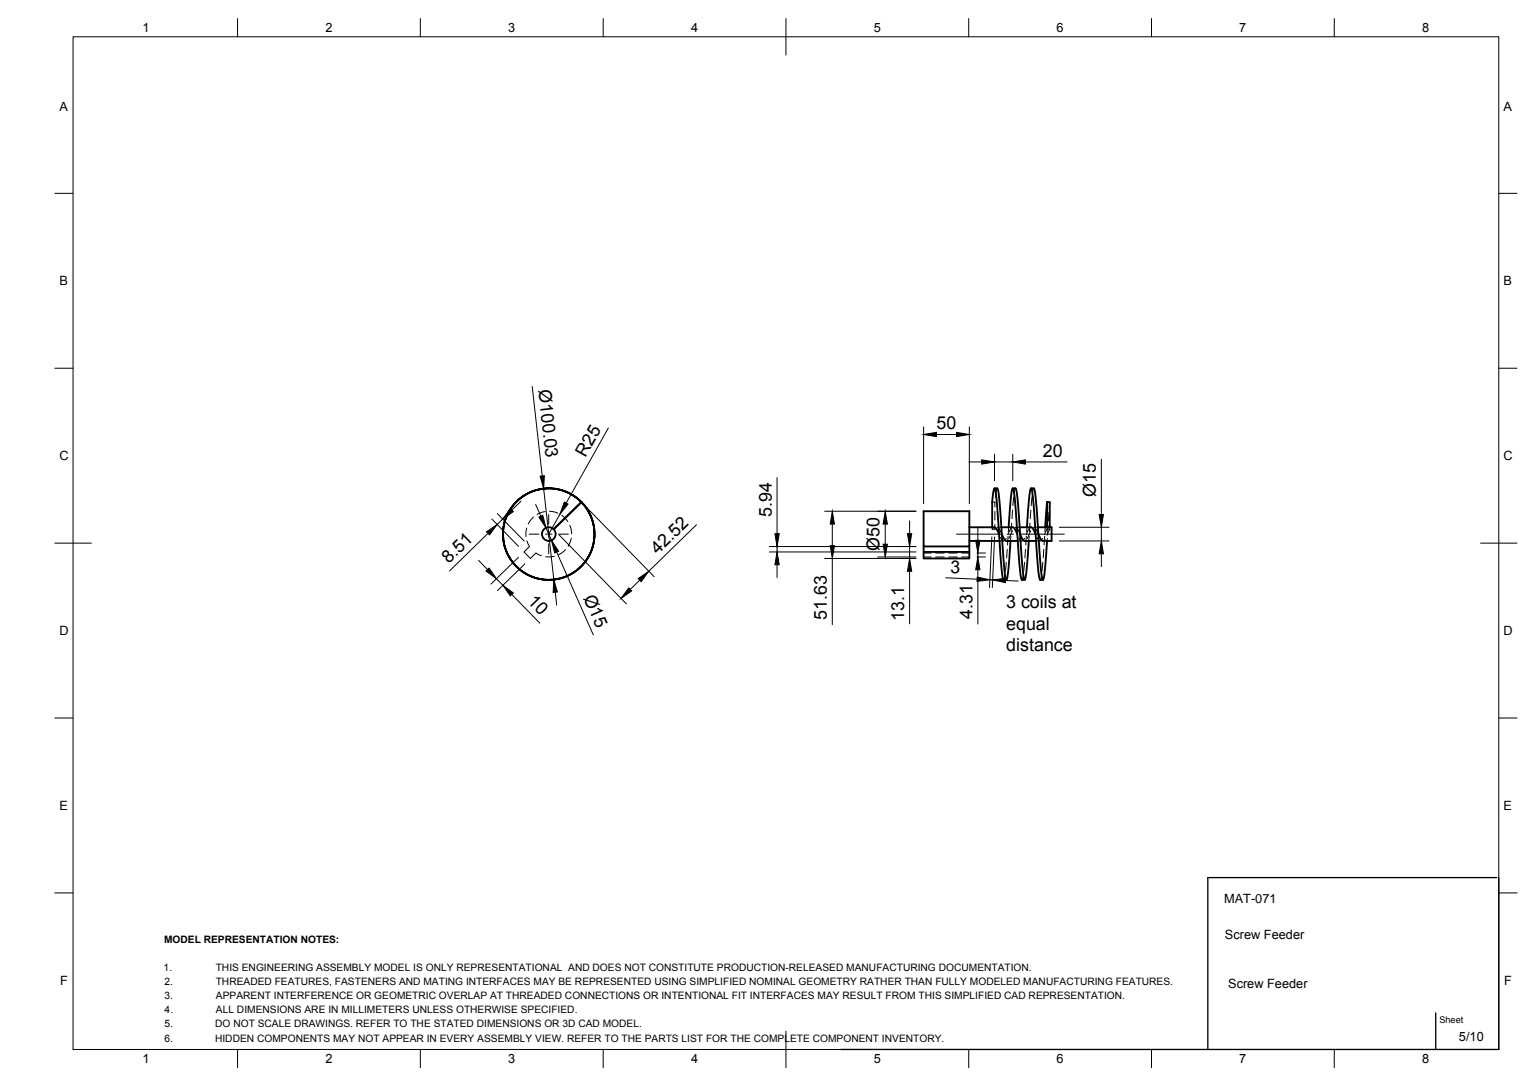
ISO-10303-21;
HEADER;
/* Generated by software containing ST-Developer
 * from STEP Tools, Inc. (www.steptools.com) 
 */

FILE_DESCRIPTION(
/* description */ (''),
/* implementation_level */ '2;1');

FILE_NAME(
/* name */ 'Screw Feeder.step',
/* time_stamp */ '2026-10-24T12:24:47-07:00',
/* author */ (''),
/* organization */ (''),
/* preprocessor_version */ 'ST-DEVELOPER v20.2',
/* originating_system */ 'Autodesk Translation Framework v15.15.0.0',
/* authorisation */ '');

FILE_SCHEMA (('AUTOMOTIVE_DESIGN { 1 0 10303 214 3 1 1 }'));
ENDSEC;

DATA;
#10=MECHANICAL_DESIGN_GEOMETRIC_PRESENTATION_REPRESENTATION('',(#62),#13594);
#50=SHAPE_REPRESENTATION_RELATIONSHIP('SRR','None',#13630,#56);
#56=ADVANCED_BREP_SHAPE_REPRESENTATION('',(#68),#13593);
#62=STYLED_ITEM('',(#13667),#68);
#68=MANIFOLD_SOLID_BREP('Screw Feeder',#2969);
#71=(
BOUNDED_SURFACE()
B_SPLINE_SURFACE(1,2,((#12578,#12579,#12580,#12581,#12582,#12583,#12584,
#12585,#12586,#12587,#12588,#12589,#12590,#12591,#12592,#12593,#12594,#12595,
#12596,#12597,#12598,#12599,#12600,#12601,#12602,#12603,#12604,#12605,#12606,
#12607,#12608,#12609,#12610,#12611,#12612,#12613,#12614,#12615,#12616,#12617,
#12618,#12619,#12620,#12621,#12622,#12623,#12624,#12625,#12626,#12627,#12628,
#12629,#12630,#12631,#12632,#12633,#12634,#12635,#12636,#12637,#12638,#12639,
#12640,#12641,#12642,#12643,#12644,#12645,#12646,#12647,#12648,#12649,#12650,
#12651,#12652,#12653,#12654,#12655,#12656,#12657,#12658,#12659,#12660,#12661,
#12662,#12663,#12664,#12665,#12666,#12667,#12668,#12669,#12670,#12671,#12672,
#12673,#12674,#12675,#12676,#12677,#12678,#12679,#12680,#12681,#12682,#12683,
#12684,#12685,#12686,#12687,#12688,#12689,#12690,#12691,#12692,#12693,#12694,
#12695,#12696,#12697,#12698),(#12699,#12700,#12701,#12702,#12703,#12704,
#12705,#12706,#12707,#12708,#12709,#12710,#12711,#12712,#12713,#12714,#12715,
#12716,#12717,#12718,#12719,#12720,#12721,#12722,#12723,#12724,#12725,#12726,
#12727,#12728,#12729,#12730,#12731,#12732,#12733,#12734,#12735,#12736,#12737,
#12738,#12739,#12740,#12741,#12742,#12743,#12744,#12745,#12746,#12747,#12748,
#12749,#12750,#12751,#12752,#12753,#12754,#12755,#12756,#12757,#12758,#12759,
#12760,#12761,#12762,#12763,#12764,#12765,#12766,#12767,#12768,#12769,#12770,
#12771,#12772,#12773,#12774,#12775,#12776,#12777,#12778,#12779,#12780,#12781,
#12782,#12783,#12784,#12785,#12786,#12787,#12788,#12789,#12790,#12791,#12792,
#12793,#12794,#12795,#12796,#12797,#12798,#12799,#12800,#12801,#12802,#12803,
#12804,#12805,#12806,#12807,#12808,#12809,#12810,#12811,#12812,#12813,#12814,
#12815,#12816,#12817,#12818,#12819)),.UNSPECIFIED.,.F.,.F.,.F.)
B_SPLINE_SURFACE_WITH_KNOTS((2,2),(3,2,2,2,2,2,2,2,2,2,2,2,2,2,2,2,2,2,
2,2,2,2,2,2,2,2,2,2,2,2,2,2,2,2,2,2,2,2,2,2,2,2,2,2,2,2,2,2,2,2,2,2,2,2,
2,2,2,2,2,2,3),(0.,1.),(0.,0.0166666666666667,0.0333333333333333,0.05,0.0666666666666667,
0.0833333333333333,0.1,0.116666666666667,0.133333333333333,0.15,0.166666666666667,
0.183333333333333,0.2,0.216666666666667,0.233333333333333,0.25,0.266666666666667,
0.283333333333333,0.3,0.316666666666667,0.333333333333333,0.35,0.366666666666667,
0.383333333333333,0.4,0.416666666666667,0.433333333333333,0.45,0.466666666666667,
0.483333333333333,0.5,0.516666666666667,0.533333333333333,0.55,0.566666666666667,
0.583333333333333,0.6,0.616666666666667,0.633333333333333,0.65,0.666666666666667,
0.683333333333333,0.7,0.716666666666667,0.733333333333333,0.75,0.766666666666667,
0.783333333333333,0.8,0.816666666666667,0.833333333333333,0.85,0.866666666666667,
0.883333333333333,0.9,0.916666666666667,0.933333333333333,0.95,0.966666666666667,
0.983333333333333,1.),.UNSPECIFIED.)
GEOMETRIC_REPRESENTATION_ITEM()
RATIONAL_B_SPLINE_SURFACE(((1.,0.987688340595138,1.,0.987688340595138,1.,
0.987688340595138,1.,0.987688340595138,1.,0.987688340595138,1.,0.987688340595138,
1.,0.987688340595138,1.,0.987688340595138,1.,0.987688340595138,1.,0.987688340595138,
1.,0.987688340595138,1.,0.987688340595138,1.,0.987688340595138,1.,0.987688340595138,
1.,0.987688340595138,1.,0.987688340595138,1.,0.987688340595138,1.,0.987688340595138,
1.,0.987688340595138,1.,0.987688340595138,1.,0.987688340595138,1.,0.987688340595138,
1.,0.987688340595138,1.,0.987688340595138,1.,0.987688340595138,1.,0.987688340595138,
1.,0.987688340595138,1.,0.987688340595138,1.,0.987688340595138,1.,0.987688340595138,
1.,0.987688340595138,1.,0.987688340595138,1.,0.987688340595138,1.,0.987688340595138,
1.,0.987688340595138,1.,0.987688340595138,1.,0.987688340595138,1.,0.987688340595138,
1.,0.987688340595138,1.,0.987688340595138,1.,0.987688340595138,1.,0.987688340595138,
1.,0.987688340595138,1.,0.987688340595138,1.,0.987688340595138,1.,0.987688340595138,
1.,0.987688340595138,1.,0.987688340595138,1.,0.987688340595138,1.,0.987688340595138,
1.,0.987688340595138,1.,0.987688340595138,1.,0.987688340595138,1.,0.987688340595138,
1.,0.987688340595138,1.,0.987688340595138,1.,0.987688340595138,1.,0.987688340595138,
1.,0.987688340595138,1.,0.987688340595138,1.),(1.,0.987688340595138,1.,
0.987688340595138,1.,0.987688340595138,1.,0.987688340595138,1.,0.987688340595138,
1.,0.987688340595138,1.,0.987688340595138,1.,0.987688340595138,1.,0.987688340595138,
1.,0.987688340595138,1.,0.987688340595138,1.,0.987688340595138,1.,0.987688340595138,
1.,0.987688340595138,1.,0.987688340595138,1.,0.987688340595138,1.,0.987688340595138,
1.,0.987688340595138,1.,0.987688340595138,1.,0.987688340595138,1.,0.987688340595138,
1.,0.987688340595138,1.,0.987688340595138,1.,0.987688340595138,1.,0.987688340595138,
1.,0.987688340595138,1.,0.987688340595138,1.,0.987688340595138,1.,0.987688340595138,
1.,0.987688340595138,1.,0.987688340595138,1.,0.987688340595138,1.,0.987688340595138,
1.,0.987688340595138,1.,0.987688340595138,1.,0.987688340595138,1.,0.987688340595138,
1.,0.987688340595138,1.,0.987688340595138,1.,0.987688340595138,1.,0.987688340595138,
1.,0.987688340595138,1.,0.987688340595138,1.,0.987688340595138,1.,0.987688340595138,
1.,0.987688340595138,1.,0.987688340595138,1.,0.987688340595138,1.,0.987688340595138,
1.,0.987688340595138,1.,0.987688340595138,1.,0.987688340595138,1.,0.987688340595138,
1.,0.987688340595138,1.,0.987688340595138,1.,0.987688340595138,1.,0.987688340595138,
1.,0.987688340595138,1.,0.987688340595138,1.,0.987688340595138,1.)))
REPRESENTATION_ITEM('')
SURFACE()
);
#72=(
BOUNDED_SURFACE()
B_SPLINE_SURFACE(1,2,((#12941,#12942,#12943,#12944,#12945,#12946,#12947,
#12948,#12949,#12950,#12951,#12952,#12953,#12954,#12955,#12956,#12957,#12958,
#12959,#12960,#12961,#12962,#12963,#12964,#12965,#12966,#12967,#12968,#12969,
#12970,#12971,#12972,#12973,#12974,#12975,#12976,#12977,#12978,#12979,#12980,
#12981,#12982,#12983,#12984,#12985,#12986,#12987,#12988,#12989,#12990,#12991,
#12992,#12993,#12994,#12995,#12996,#12997,#12998,#12999,#13000,#13001,#13002,
#13003,#13004,#13005,#13006,#13007,#13008,#13009,#13010,#13011,#13012,#13013,
#13014,#13015,#13016,#13017,#13018,#13019,#13020,#13021,#13022,#13023,#13024,
#13025,#13026,#13027,#13028,#13029,#13030,#13031,#13032,#13033,#13034,#13035,
#13036,#13037,#13038,#13039,#13040,#13041,#13042,#13043,#13044,#13045,#13046,
#13047,#13048,#13049,#13050,#13051,#13052,#13053,#13054,#13055,#13056,#13057,
#13058,#13059,#13060,#13061),(#13062,#13063,#13064,#13065,#13066,#13067,
#13068,#13069,#13070,#13071,#13072,#13073,#13074,#13075,#13076,#13077,#13078,
#13079,#13080,#13081,#13082,#13083,#13084,#13085,#13086,#13087,#13088,#13089,
#13090,#13091,#13092,#13093,#13094,#13095,#13096,#13097,#13098,#13099,#13100,
#13101,#13102,#13103,#13104,#13105,#13106,#13107,#13108,#13109,#13110,#13111,
#13112,#13113,#13114,#13115,#13116,#13117,#13118,#13119,#13120,#13121,#13122,
#13123,#13124,#13125,#13126,#13127,#13128,#13129,#13130,#13131,#13132,#13133,
#13134,#13135,#13136,#13137,#13138,#13139,#13140,#13141,#13142,#13143,#13144,
#13145,#13146,#13147,#13148,#13149,#13150,#13151,#13152,#13153,#13154,#13155,
#13156,#13157,#13158,#13159,#13160,#13161,#13162,#13163,#13164,#13165,#13166,
#13167,#13168,#13169,#13170,#13171,#13172,#13173,#13174,#13175,#13176,#13177,
#13178,#13179,#13180,#13181,#13182)),.UNSPECIFIED.,.F.,.F.,.F.)
B_SPLINE_SURFACE_WITH_KNOTS((2,2),(3,2,2,2,2,2,2,2,2,2,2,2,2,2,2,2,2,2,
2,2,2,2,2,2,2,2,2,2,2,2,2,2,2,2,2,2,2,2,2,2,2,2,2,2,2,2,2,2,2,2,2,2,2,2,
2,2,2,2,2,2,3),(0.,1.),(0.,0.0166666666666667,0.0333333333333333,0.05,0.0666666666666667,
0.0833333333333333,0.1,0.116666666666667,0.133333333333333,0.15,0.166666666666667,
0.183333333333333,0.2,0.216666666666667,0.233333333333333,0.25,0.266666666666667,
0.283333333333333,0.3,0.316666666666667,0.333333333333333,0.35,0.366666666666667,
0.383333333333333,0.4,0.416666666666667,0.433333333333333,0.45,0.466666666666667,
0.483333333333333,0.5,0.516666666666667,0.533333333333333,0.55,0.566666666666667,
0.583333333333333,0.6,0.616666666666667,0.633333333333333,0.65,0.666666666666667,
0.683333333333333,0.7,0.716666666666667,0.733333333333333,0.75,0.766666666666667,
0.783333333333333,0.8,0.816666666666667,0.833333333333333,0.85,0.866666666666667,
0.883333333333333,0.9,0.916666666666667,0.933333333333333,0.95,0.966666666666667,
0.983333333333333,1.),.UNSPECIFIED.)
GEOMETRIC_REPRESENTATION_ITEM()
RATIONAL_B_SPLINE_SURFACE(((1.,0.987688340595138,1.,0.987688340595138,1.,
0.987688340595138,1.,0.987688340595138,1.,0.987688340595138,1.,0.987688340595138,
1.,0.987688340595138,1.,0.987688340595138,1.,0.987688340595138,1.,0.987688340595138,
1.,0.987688340595138,1.,0.987688340595138,1.,0.987688340595138,1.,0.987688340595138,
1.,0.987688340595138,1.,0.987688340595138,1.,0.987688340595138,1.,0.987688340595138,
1.,0.987688340595138,1.,0.987688340595138,1.,0.987688340595138,1.,0.987688340595138,
1.,0.987688340595138,1.,0.987688340595138,1.,0.987688340595138,1.,0.987688340595138,
1.,0.987688340595138,1.,0.987688340595138,1.,0.987688340595138,1.,0.987688340595138,
1.,0.987688340595138,1.,0.987688340595138,1.,0.987688340595138,1.,0.987688340595138,
1.,0.987688340595138,1.,0.987688340595138,1.,0.987688340595138,1.,0.987688340595138,
1.,0.987688340595138,1.,0.987688340595138,1.,0.987688340595138,1.,0.987688340595138,
1.,0.987688340595138,1.,0.987688340595138,1.,0.987688340595138,1.,0.987688340595138,
1.,0.987688340595138,1.,0.987688340595138,1.,0.987688340595138,1.,0.987688340595138,
1.,0.987688340595138,1.,0.987688340595138,1.,0.987688340595138,1.,0.987688340595138,
1.,0.987688340595138,1.,0.987688340595138,1.,0.987688340595138,1.,0.987688340595138,
1.,0.987688340595138,1.,0.987688340595138,1.),(1.,0.987688340595138,1.,
0.987688340595138,1.,0.987688340595138,1.,0.987688340595138,1.,0.987688340595138,
1.,0.987688340595138,1.,0.987688340595138,1.,0.987688340595138,1.,0.987688340595138,
1.,0.987688340595138,1.,0.987688340595138,1.,0.987688340595138,1.,0.987688340595138,
1.,0.987688340595138,1.,0.987688340595138,1.,0.987688340595138,1.,0.987688340595138,
1.,0.987688340595138,1.,0.987688340595138,1.,0.987688340595138,1.,0.987688340595138,
1.,0.987688340595138,1.,0.987688340595138,1.,0.987688340595138,1.,0.987688340595138,
1.,0.987688340595138,1.,0.987688340595138,1.,0.987688340595138,1.,0.987688340595138,
1.,0.987688340595138,1.,0.987688340595138,1.,0.987688340595138,1.,0.987688340595138,
1.,0.987688340595138,1.,0.987688340595138,1.,0.987688340595138,1.,0.987688340595138,
1.,0.987688340595138,1.,0.987688340595138,1.,0.987688340595138,1.,0.987688340595138,
1.,0.987688340595138,1.,0.987688340595138,1.,0.987688340595138,1.,0.987688340595138,
1.,0.987688340595138,1.,0.987688340595138,1.,0.987688340595138,1.,0.987688340595138,
1.,0.987688340595138,1.,0.987688340595138,1.,0.987688340595138,1.,0.987688340595138,
1.,0.987688340595138,1.,0.987688340595138,1.,0.987688340595138,1.,0.987688340595138,
1.,0.987688340595138,1.,0.987688340595138,1.,0.987688340595138,1.)))
REPRESENTATION_ITEM('')
SURFACE()
);
#73=(
BOUNDED_SURFACE()
B_SPLINE_SURFACE(1,2,((#13304,#13305,#13306,#13307,#13308,#13309,#13310,
#13311,#13312,#13313,#13314,#13315,#13316,#13317,#13318,#13319,#13320,#13321,
#13322,#13323,#13324,#13325,#13326,#13327,#13328,#13329,#13330,#13331,#13332,
#13333,#13334,#13335,#13336,#13337,#13338,#13339,#13340,#13341,#13342,#13343,
#13344,#13345,#13346,#13347,#13348,#13349,#13350,#13351,#13352,#13353,#13354,
#13355,#13356,#13357,#13358,#13359,#13360,#13361,#13362,#13363,#13364,#13365,
#13366,#13367,#13368,#13369,#13370,#13371,#13372,#13373,#13374,#13375,#13376,
#13377,#13378,#13379,#13380,#13381,#13382,#13383,#13384,#13385,#13386,#13387,
#13388,#13389,#13390,#13391,#13392,#13393,#13394,#13395,#13396,#13397,#13398,
#13399,#13400,#13401,#13402,#13403,#13404,#13405,#13406,#13407,#13408,#13409,
#13410,#13411,#13412,#13413,#13414,#13415,#13416,#13417,#13418,#13419,#13420,
#13421,#13422,#13423,#13424),(#13425,#13426,#13427,#13428,#13429,#13430,
#13431,#13432,#13433,#13434,#13435,#13436,#13437,#13438,#13439,#13440,#13441,
#13442,#13443,#13444,#13445,#13446,#13447,#13448,#13449,#13450,#13451,#13452,
#13453,#13454,#13455,#13456,#13457,#13458,#13459,#13460,#13461,#13462,#13463,
#13464,#13465,#13466,#13467,#13468,#13469,#13470,#13471,#13472,#13473,#13474,
#13475,#13476,#13477,#13478,#13479,#13480,#13481,#13482,#13483,#13484,#13485,
#13486,#13487,#13488,#13489,#13490,#13491,#13492,#13493,#13494,#13495,#13496,
#13497,#13498,#13499,#13500,#13501,#13502,#13503,#13504,#13505,#13506,#13507,
#13508,#13509,#13510,#13511,#13512,#13513,#13514,#13515,#13516,#13517,#13518,
#13519,#13520,#13521,#13522,#13523,#13524,#13525,#13526,#13527,#13528,#13529,
#13530,#13531,#13532,#13533,#13534,#13535,#13536,#13537,#13538,#13539,#13540,
#13541,#13542,#13543,#13544,#13545)),.UNSPECIFIED.,.F.,.F.,.F.)
B_SPLINE_SURFACE_WITH_KNOTS((2,2),(3,2,2,2,2,2,2,2,2,2,2,2,2,2,2,2,2,2,
2,2,2,2,2,2,2,2,2,2,2,2,2,2,2,2,2,2,2,2,2,2,2,2,2,2,2,2,2,2,2,2,2,2,2,2,
2,2,2,2,2,2,3),(0.,1.),(0.,0.0166666666666667,0.0333333333333333,0.05,0.0666666666666667,
0.0833333333333333,0.1,0.116666666666667,0.133333333333333,0.15,0.166666666666667,
0.183333333333333,0.2,0.216666666666667,0.233333333333333,0.25,0.266666666666667,
0.283333333333333,0.3,0.316666666666667,0.333333333333333,0.35,0.366666666666667,
0.383333333333333,0.4,0.416666666666667,0.433333333333333,0.45,0.466666666666667,
0.483333333333333,0.5,0.516666666666667,0.533333333333333,0.55,0.566666666666667,
0.583333333333333,0.6,0.616666666666667,0.633333333333333,0.65,0.666666666666667,
0.683333333333333,0.7,0.716666666666667,0.733333333333333,0.75,0.766666666666667,
0.783333333333333,0.8,0.816666666666667,0.833333333333333,0.85,0.866666666666667,
0.883333333333333,0.9,0.916666666666667,0.933333333333333,0.95,0.966666666666667,
0.983333333333333,1.),.UNSPECIFIED.)
GEOMETRIC_REPRESENTATION_ITEM()
RATIONAL_B_SPLINE_SURFACE(((1.,0.987688340595138,1.,0.987688340595138,1.,
0.987688340595138,1.,0.987688340595138,1.,0.987688340595138,1.,0.987688340595138,
1.,0.987688340595138,1.,0.987688340595138,1.,0.987688340595138,1.,0.987688340595138,
1.,0.987688340595138,1.,0.987688340595138,1.,0.987688340595138,1.,0.987688340595138,
1.,0.987688340595138,1.,0.987688340595138,1.,0.987688340595138,1.,0.987688340595138,
1.,0.987688340595138,1.,0.987688340595138,1.,0.987688340595138,1.,0.987688340595138,
1.,0.987688340595138,1.,0.987688340595138,1.,0.987688340595138,1.,0.987688340595138,
1.,0.987688340595138,1.,0.987688340595138,1.,0.987688340595138,1.,0.987688340595138,
1.,0.987688340595138,1.,0.987688340595138,1.,0.987688340595138,1.,0.987688340595138,
1.,0.987688340595138,1.,0.987688340595138,1.,0.987688340595138,1.,0.987688340595138,
1.,0.987688340595138,1.,0.987688340595138,1.,0.987688340595138,1.,0.987688340595138,
1.,0.987688340595138,1.,0.987688340595138,1.,0.987688340595138,1.,0.987688340595138,
1.,0.987688340595138,1.,0.987688340595138,1.,0.987688340595138,1.,0.987688340595138,
1.,0.987688340595138,1.,0.987688340595138,1.,0.987688340595138,1.,0.987688340595138,
1.,0.987688340595138,1.,0.987688340595138,1.,0.987688340595138,1.,0.987688340595138,
1.,0.987688340595138,1.,0.987688340595138,1.),(1.,0.987688340595138,1.,
0.987688340595138,1.,0.987688340595138,1.,0.987688340595138,1.,0.987688340595138,
1.,0.987688340595138,1.,0.987688340595138,1.,0.987688340595138,1.,0.987688340595138,
1.,0.987688340595138,1.,0.987688340595138,1.,0.987688340595138,1.,0.987688340595138,
1.,0.987688340595138,1.,0.987688340595138,1.,0.987688340595138,1.,0.987688340595138,
1.,0.987688340595138,1.,0.987688340595138,1.,0.987688340595138,1.,0.987688340595138,
1.,0.987688340595138,1.,0.987688340595138,1.,0.987688340595138,1.,0.987688340595138,
1.,0.987688340595138,1.,0.987688340595138,1.,0.987688340595138,1.,0.987688340595138,
1.,0.987688340595138,1.,0.987688340595138,1.,0.987688340595138,1.,0.987688340595138,
1.,0.987688340595138,1.,0.987688340595138,1.,0.987688340595138,1.,0.987688340595138,
1.,0.987688340595138,1.,0.987688340595138,1.,0.987688340595138,1.,0.987688340595138,
1.,0.987688340595138,1.,0.987688340595138,1.,0.987688340595138,1.,0.987688340595138,
1.,0.987688340595138,1.,0.987688340595138,1.,0.987688340595138,1.,0.987688340595138,
1.,0.987688340595138,1.,0.987688340595138,1.,0.987688340595138,1.,0.987688340595138,
1.,0.987688340595138,1.,0.987688340595138,1.,0.987688340595138,1.,0.987688340595138,
1.,0.987688340595138,1.,0.987688340595138,1.,0.987688340595138,1.)))
REPRESENTATION_ITEM('')
SURFACE()
);
#104=PLANE('',#3260);
#105=PLANE('',#3261);
#106=PLANE('',#3262);
#107=PLANE('',#3266);
#108=PLANE('',#3267);
#109=PLANE('',#3268);
#110=PLANE('',#3269);
#111=PLANE('',#3270);
#134=FACE_BOUND('',#568,.T.);
#143=B_SPLINE_CURVE_WITH_KNOTS('',3,(#11375,#11376,#11377,#11378),
 .UNSPECIFIED.,.F.,.F.,(4,4),(-1.,-0.998645968698766),.UNSPECIFIED.);
#144=B_SPLINE_CURVE_WITH_KNOTS('',3,(#11385,#11386,#11387,#11388,#11389,
#11390,#11391,#11392,#11393,#11394,#11395,#11396,#11397,#11398,#11399,#11400,
#11401,#11402,#11403,#11404,#11405,#11406,#11407,#11408,#11409,#11410,#11411,
#11412,#11413,#11414,#11415,#11416,#11417,#11418,#11419,#11420,#11421,#11422,
#11423,#11424,#11425,#11426,#11427,#11428,#11429,#11430,#11431,#11432,#11433,
#11434,#11435,#11436,#11437,#11438,#11439,#11440,#11441,#11442,#11443,#11444,
#11445,#11446,#11447,#11448,#11449,#11450,#11451,#11452,#11453,#11454,#11455,
#11456,#11457,#11458,#11459,#11460,#11461,#11462,#11463,#11464,#11465,#11466,
#11467,#11468,#11469,#11470,#11471,#11472,#11473,#11474,#11475,#11476,#11477,
#11478,#11479,#11480,#11481,#11482,#11483,#11484,#11485,#11486,#11487,#11488,
#11489,#11490,#11491,#11492,#11493,#11494,#11495,#11496,#11497,#11498,#11499,
#11500,#11501,#11502,#11503,#11504,#11505,#11506,#11507,#11508,#11509,#11510,
#11511,#11512,#11513,#11514,#11515,#11516,#11517,#11518,#11519,#11520,#11521,
#11522,#11523,#11524,#11525,#11526,#11527,#11528,#11529,#11530,#11531,#11532,
#11533,#11534,#11535,#11536,#11537,#11538,#11539,#11540,#11541,#11542,#11543,
#11544,#11545,#11546,#11547,#11548,#11549,#11550,#11551,#11552,#11553,#11554,
#11555,#11556,#11557,#11558,#11559,#11560,#11561,#11562,#11563,#11564,#11565,
#11566,#11567,#11568,#11569,#11570,#11571,#11572,#11573,#11574,#11575,#11576,
#11577,#11578,#11579,#11580,#11581,#11582,#11583,#11584,#11585,#11586,#11587,
#11588,#11589,#11590,#11591,#11592,#11593,#11594,#11595,#11596,#11597,#11598,
#11599,#11600,#11601,#11602,#11603,#11604,#11605,#11606,#11607,#11608,#11609,
#11610,#11611,#11612,#11613,#11614,#11615,#11616,#11617,#11618,#11619,#11620,
#11621,#11622,#11623,#11624,#11625,#11626,#11627,#11628,#11629,#11630,#11631,
#11632,#11633,#11634,#11635,#11636,#11637,#11638,#11639,#11640,#11641,#11642,
#11643,#11644,#11645,#11646,#11647,#11648,#11649,#11650,#11651,#11652,#11653,
#11654,#11655,#11656,#11657,#11658,#11659,#11660,#11661,#11662,#11663,#11664,
#11665,#11666,#11667,#11668,#11669,#11670,#11671,#11672,#11673,#11674,#11675,
#11676,#11677,#11678,#11679,#11680,#11681,#11682,#11683,#11684,#11685,#11686,
#11687,#11688,#11689,#11690,#11691,#11692,#11693,#11694,#11695,#11696,#11697,
#11698,#11699,#11700,#11701,#11702,#11703,#11704,#11705,#11706,#11707,#11708,
#11709,#11710,#11711,#11712,#11713,#11714,#11715,#11716,#11717,#11718,#11719,
#11720,#11721,#11722,#11723,#11724,#11725,#11726,#11727,#11728,#11729,#11730,
#11731,#11732,#11733,#11734,#11735,#11736,#11737,#11738,#11739,#11740,#11741,
#11742),.UNSPECIFIED.,.F.,.F.,(4,3,3,3,3,3,3,3,3,3,3,3,3,3,3,3,3,3,3,3,
3,3,3,3,3,3,3,3,3,3,3,3,3,3,3,3,3,3,3,3,3,3,3,3,3,3,3,3,3,3,3,3,3,3,3,3,
3,3,3,3,3,3,3,3,3,3,3,3,3,3,3,3,3,3,3,3,3,3,3,3,3,3,3,3,3,3,3,3,3,3,3,3,
3,3,3,3,3,3,3,3,3,3,3,3,3,3,3,3,3,3,3,3,3,3,3,3,3,3,3,4),(-0.331979302032099,
-0.328745544947817,-0.325511126349503,-0.322277581756429,-0.319042795051795,
-0.316666666666667,-0.313432410645245,-0.310074307983934,-0.306840488099785,
-0.303607230746873,-0.300373105768056,-0.3,-0.296765743978578,-0.293407641317267,
-0.290173821433118,-0.286940564080179,-0.283706439101408,-0.283333333333333,
-0.280099077311897,-0.27674097465059,-0.273507154766441,-0.270273897413541,
-0.267039772434759,-0.266666666666667,-0.263432410645244,-0.260074307983933,
-0.25684048809978,-0.253607230746841,-0.250373105768036,-0.25,-0.246765743978575,
-0.243407641317264,-0.240173821433105,-0.236940564080198,-0.233706439101398,
-0.233333333333333,-0.230099077311924,-0.22674097465061,-0.223507154766454,
-0.220273897413536,-0.217039772434708,-0.216666666666667,-0.213432410645268,
-0.210074307983951,-0.206840488099798,-0.203607230746877,-0.200373105768084,
-0.2,-0.196765743978578,-0.193407641317267,-0.190173821433123,-0.186940564080229,
-0.183706439101414,-0.183333333333333,-0.180099077311908,-0.176740974650597,
-0.173507154766428,-0.170273897413483,-0.167039772434678,-0.166666666666667,
-0.163432410645259,-0.160074307983944,-0.156840488099797,-0.153607230746853,
-0.150373105768069,-0.15,-0.146765743978574,-0.143407641317264,-0.140173821433101,
-0.136940564080169,-0.133706439101386,-0.133333333333333,-0.130099077311911,
-0.1267409746506,-0.123507154766447,-0.120273897413526,-0.117039772434722,
-0.116666666666667,-0.113432410645241,-0.110074307983931,-0.106840488099774,
-0.103607230746858,-0.10037310576804,-0.1,-0.0967657439785776,-0.0934076413172665,
-0.0901738214331063,-0.0869405640801917,-0.0837064391013879,-0.0833333333333334,
-0.0800990773119075,-0.0767409746505973,-0.0735071547664396,-0.0702738974135466,
-0.0670397724347522,-0.0666666666666667,-0.0634324106452447,-0.0600743079839336,
-0.0568404880997839,-0.0536072307468639,-0.0503731057680767,-0.05,-0.0467657439785748,
-0.0434076413172644,-0.0401738214331216,-0.0369405640801967,-0.033706439101418,
-0.0333333333333333,-0.030099077311911,-0.0267409746505999,-0.0235071547664523,
-0.0202738974135343,-0.017039772434738,-0.0166666666666667,-0.0134324106517174,
-0.0100743318149406,-0.00684051195133032,-0.00360725461687006,-0.000373129688631168,
-9.53046099950368E-8),.UNSPECIFIED.);
#145=B_SPLINE_CURVE_WITH_KNOTS('',3,(#11789,#11790,#11791,#11792,#11793,
#11794,#11795,#11796,#11797,#11798,#11799,#11800,#11801,#11802,#11803,#11804,
#11805,#11806,#11807,#11808,#11809,#11810,#11811,#11812,#11813,#11814,#11815,
#11816,#11817,#11818,#11819,#11820,#11821,#11822,#11823,#11824,#11825,#11826,
#11827,#11828,#11829,#11830,#11831,#11832,#11833,#11834,#11835,#11836,#11837,
#11838,#11839,#11840,#11841,#11842,#11843,#11844,#11845,#11846,#11847,#11848,
#11849,#11850,#11851,#11852,#11853,#11854,#11855,#11856,#11857,#11858,#11859,
#11860,#11861,#11862,#11863,#11864,#11865,#11866,#11867,#11868,#11869,#11870,
#11871,#11872,#11873,#11874,#11875,#11876,#11877,#11878,#11879,#11880,#11881,
#11882,#11883,#11884,#11885,#11886,#11887,#11888,#11889,#11890,#11891,#11892,
#11893,#11894,#11895,#11896,#11897,#11898,#11899,#11900,#11901,#11902,#11903,
#11904,#11905,#11906,#11907,#11908,#11909,#11910,#11911,#11912,#11913,#11914,
#11915,#11916,#11917,#11918,#11919,#11920,#11921,#11922,#11923,#11924,#11925,
#11926,#11927,#11928,#11929,#11930,#11931,#11932,#11933,#11934,#11935,#11936,
#11937,#11938,#11939,#11940,#11941,#11942,#11943,#11944,#11945,#11946,#11947,
#11948,#11949,#11950,#11951,#11952,#11953,#11954,#11955,#11956,#11957,#11958,
#11959,#11960,#11961,#11962,#11963,#11964,#11965,#11966,#11967,#11968,#11969,
#11970,#11971,#11972,#11973,#11974,#11975,#11976,#11977,#11978,#11979,#11980,
#11981,#11982,#11983,#11984,#11985,#11986,#11987,#11988,#11989,#11990,#11991,
#11992,#11993,#11994,#11995,#11996,#11997,#11998,#11999,#12000,#12001,#12002,
#12003,#12004,#12005,#12006,#12007,#12008,#12009,#12010,#12011,#12012,#12013,
#12014,#12015,#12016,#12017,#12018,#12019,#12020,#12021,#12022,#12023,#12024,
#12025,#12026,#12027,#12028,#12029,#12030,#12031,#12032,#12033,#12034,#12035,
#12036,#12037,#12038,#12039,#12040,#12041,#12042,#12043,#12044,#12045,#12046,
#12047,#12048,#12049,#12050,#12051,#12052,#12053,#12054,#12055,#12056,#12057,
#12058,#12059,#12060,#12061,#12062,#12063,#12064,#12065,#12066,#12067,#12068,
#12069,#12070,#12071,#12072,#12073,#12074,#12075,#12076,#12077,#12078,#12079,
#12080,#12081,#12082,#12083,#12084,#12085,#12086,#12087,#12088,#12089,#12090,
#12091,#12092,#12093,#12094,#12095,#12096,#12097,#12098,#12099,#12100,#12101,
#12102,#12103,#12104,#12105,#12106,#12107,#12108,#12109,#12110,#12111,#12112,
#12113,#12114,#12115,#12116,#12117,#12118,#12119,#12120,#12121,#12122,#12123,
#12124,#12125,#12126,#12127,#12128,#12129,#12130,#12131,#12132,#12133,#12134,
#12135,#12136,#12137,#12138,#12139,#12140,#12141,#12142,#12143,#12144,#12145,
#12146,#12147,#12148,#12149),.UNSPECIFIED.,.F.,.F.,(4,3,3,3,3,3,3,3,3,3,
3,3,3,3,3,3,3,3,3,3,3,3,3,3,3,3,3,3,3,3,3,3,3,3,3,3,3,3,3,3,3,3,3,3,3,3,
3,3,3,3,3,3,3,3,3,3,3,3,3,3,3,3,3,3,3,3,3,3,3,3,3,3,3,3,3,3,3,3,3,3,3,3,
3,3,3,3,3,3,3,3,3,3,3,3,3,3,3,3,3,3,3,3,3,3,3,3,3,3,3,3,3,3,3,3,3,3,3,3,
3,3,4),(-0.665312635365433,-0.662078878281142,-0.658844459682826,-0.655610915089758,
-0.652376128385123,-0.65,-0.646765743978579,-0.643407641317267,-0.640173821433118,
-0.636940564080195,-0.633706439101402,-0.633333333333333,-0.630099077311912,
-0.626740974650601,-0.623507154766448,-0.620273897413523,-0.617039772434729,
-0.616666666666667,-0.613432410645243,-0.610074307983932,-0.60684048809978,
-0.603607230746855,-0.60037310576806,-0.6,-0.596765743978578,-0.593407641317267,
-0.590173821433114,-0.586940564080189,-0.583706439101395,-0.583333333333333,
-0.580099077311911,-0.5767409746506,-0.573507154766447,-0.570273897413521,
-0.567039772434727,-0.566666666666667,-0.563432410645245,-0.560074307983934,
-0.556840488099781,-0.553607230746856,-0.550373105768065,-0.55,-0.546765743978579,
-0.543407641317267,-0.540173821433115,-0.536940564080189,-0.533706439101384,
-0.533333333333333,-0.530099077311911,-0.5267409746506,-0.523507154766446,
-0.52027389741352,-0.517039772434727,-0.516666666666667,-0.513432410645245,
-0.510074307983934,-0.506840488099781,-0.503607230746855,-0.500373105768063,
-0.5,-0.496765743978578,-0.493407641317267,-0.490173821433103,-0.486940564080178,
-0.483706439101384,-0.483333333333333,-0.480099077311911,-0.4767409746506,
-0.473507154766447,-0.47027389741351,-0.467039772434717,-0.466666666666667,
-0.463432410645245,-0.460074307983933,-0.456840488099777,-0.453607230746852,
-0.450373105768059,-0.45,-0.446765743978577,-0.443407641317266,-0.440173821433109,
-0.43694056408017,-0.433706439101377,-0.433333333333333,-0.430099077311911,
-0.4267409746506,-0.423507154766447,-0.420273897413509,-0.417039772434716,
-0.416666666666667,-0.413432410645244,-0.410074307983933,-0.40684048809978,
-0.403607230746867,-0.400373105768075,-0.4,-0.396765743978578,-0.393407641317267,
-0.390173821433118,-0.386940564080206,-0.383706439101414,-0.383333333333333,
-0.380099077311912,-0.376740974650601,-0.373507154766456,-0.370273897413568,
-0.367039772434754,-0.366666666666667,-0.363432410645244,-0.360074307983933,
-0.356840488099784,-0.353607230746845,-0.350373105768042,-0.35,-0.346765743978578,
-0.343407641317267,-0.34017382143311,-0.336940564080171,-0.333706439101378,
-0.333333333333333,-0.331979302032099),.UNSPECIFIED.);
#146=B_SPLINE_CURVE_WITH_KNOTS('',3,(#12194,#12195,#12196,#12197,#12198,
#12199,#12200,#12201,#12202,#12203,#12204,#12205,#12206,#12207,#12208,#12209,
#12210,#12211,#12212,#12213,#12214,#12215,#12216,#12217,#12218,#12219,#12220,
#12221,#12222,#12223,#12224,#12225,#12226,#12227,#12228,#12229,#12230,#12231,
#12232,#12233,#12234,#12235,#12236,#12237,#12238,#12239,#12240,#12241,#12242,
#12243,#12244,#12245,#12246,#12247,#12248,#12249,#12250,#12251,#12252,#12253,
#12254,#12255,#12256,#12257,#12258,#12259,#12260,#12261,#12262,#12263,#12264,
#12265,#12266,#12267,#12268,#12269,#12270,#12271,#12272,#12273,#12274,#12275,
#12276,#12277,#12278,#12279,#12280,#12281,#12282,#12283,#12284,#12285,#12286,
#12287,#12288,#12289,#12290,#12291,#12292,#12293,#12294,#12295,#12296,#12297,
#12298,#12299,#12300,#12301,#12302,#12303,#12304,#12305,#12306,#12307,#12308,
#12309,#12310,#12311,#12312,#12313,#12314,#12315,#12316,#12317,#12318,#12319,
#12320,#12321,#12322,#12323,#12324,#12325,#12326,#12327,#12328,#12329,#12330,
#12331,#12332,#12333,#12334,#12335,#12336,#12337,#12338,#12339,#12340,#12341,
#12342,#12343,#12344,#12345,#12346,#12347,#12348,#12349,#12350,#12351,#12352,
#12353,#12354,#12355,#12356,#12357,#12358,#12359,#12360,#12361,#12362,#12363,
#12364,#12365,#12366,#12367,#12368,#12369,#12370,#12371,#12372,#12373,#12374,
#12375,#12376,#12377,#12378,#12379,#12380,#12381,#12382,#12383,#12384,#12385,
#12386,#12387,#12388,#12389,#12390,#12391,#12392,#12393,#12394,#12395,#12396,
#12397,#12398,#12399,#12400,#12401,#12402,#12403,#12404,#12405,#12406,#12407,
#12408,#12409,#12410,#12411,#12412,#12413,#12414,#12415,#12416,#12417,#12418,
#12419,#12420,#12421,#12422,#12423,#12424,#12425,#12426,#12427,#12428,#12429,
#12430,#12431,#12432,#12433,#12434,#12435,#12436,#12437,#12438,#12439,#12440,
#12441,#12442,#12443,#12444,#12445,#12446,#12447,#12448,#12449,#12450,#12451,
#12452,#12453,#12454,#12455,#12456,#12457,#12458,#12459,#12460,#12461,#12462,
#12463,#12464,#12465,#12466,#12467,#12468,#12469,#12470,#12471,#12472,#12473,
#12474,#12475,#12476,#12477,#12478,#12479,#12480,#12481,#12482,#12483,#12484,
#12485,#12486,#12487,#12488,#12489,#12490,#12491,#12492,#12493,#12494,#12495,
#12496,#12497,#12498,#12499,#12500,#12501,#12502,#12503,#12504,#12505,#12506,
#12507,#12508,#12509,#12510,#12511,#12512,#12513,#12514,#12515,#12516,#12517,
#12518,#12519,#12520,#12521,#12522,#12523,#12524,#12525,#12526,#12527,#12528,
#12529,#12530,#12531,#12532,#12533,#12534,#12535,#12536,#12537,#12538,#12539,
#12540,#12541,#12542,#12543,#12544,#12545,#12546,#12547,#12548,#12549,#12550,
#12551,#12552,#12553,#12554),.UNSPECIFIED.,.F.,.F.,(4,3,3,3,3,3,3,3,3,3,
3,3,3,3,3,3,3,3,3,3,3,3,3,3,3,3,3,3,3,3,3,3,3,3,3,3,3,3,3,3,3,3,3,3,3,3,
3,3,3,3,3,3,3,3,3,3,3,3,3,3,3,3,3,3,3,3,3,3,3,3,3,3,3,3,3,3,3,3,3,3,3,3,
3,3,3,3,3,3,3,3,3,3,3,3,3,3,3,3,3,3,3,3,3,3,3,3,3,3,3,3,3,3,3,3,3,3,3,3,
3,3,4),(-0.998645968698766,-0.995412211614476,-0.99217779301616,-0.988944248423087,
-0.985709461718452,-0.983333333333333,-0.980099077311911,-0.9767409746506,
-0.973507154766447,-0.970273897413519,-0.967039772434726,-0.966666666666667,
-0.963432410645243,-0.960074307983932,-0.956840488099779,-0.953607230746854,
-0.950373105768062,-0.95,-0.946765743978577,-0.943407641317266,-0.940173821433113,
-0.936940564080185,-0.933706439101392,-0.933333333333333,-0.930099077311911,
-0.9267409746506,-0.923507154766446,-0.92027389741352,-0.917039772434728,
-0.916666666666667,-0.913432410645244,-0.910074307983933,-0.90684048809978,
-0.903607230746854,-0.90037310576806,-0.9,-0.896765743978578,-0.893407641317267,
-0.890173821433115,-0.886940564080189,-0.883706439101396,-0.883333333333333,
-0.880099077311911,-0.8767409746506,-0.873507154766449,-0.870273897413525,
-0.867039772434733,-0.866666666666667,-0.863432410645245,-0.860074307983934,
-0.856840488099781,-0.853607230746854,-0.850373105768058,-0.85,-0.846765743978578,
-0.843407641317267,-0.840173821433114,-0.836940564080188,-0.833706439101395,
-0.833333333333333,-0.830099077311911,-0.8267409746506,-0.823507154766447,
-0.820273897413526,-0.817039772434731,-0.816666666666667,-0.81343241064524,
-0.81007430798393,-0.806840488099777,-0.803607230746853,-0.800373105768059,
-0.8,-0.796765743978579,-0.793407641317267,-0.790173821433115,-0.786940564080183,
-0.783706439101388,-0.783333333333333,-0.780099077311911,-0.7767409746506,
-0.773507154766446,-0.770273897413509,-0.767039772434712,-0.766666666666667,
-0.763432410645249,-0.760074307983936,-0.756840488099782,-0.753607230746868,
-0.75037310576807,-0.75,-0.746765743978578,-0.743407641317267,-0.740173821433118,
-0.736940564080168,-0.733706439101356,-0.733333333333333,-0.730099077311911,
-0.7267409746506,-0.723507154766451,-0.720273897413524,-0.717039772434739,
-0.716666666666667,-0.713432410645237,-0.710074307983928,-0.706840488099775,
-0.703607230746849,-0.700373105768067,-0.7,-0.69676574397857,-0.693407641317261,
-0.690173821433107,-0.686940564080183,-0.683706439101389,-0.683333333333333,
-0.680099077311912,-0.6767409746506,-0.673507154766448,-0.670273897413522,
-0.667039772434727,-0.666666666666667,-0.665312635365433),.UNSPECIFIED.);
#147=B_SPLINE_CURVE_WITH_KNOTS('',3,(#12558,#12559,#12560,#12561,#12562,
#12563),.UNSPECIFIED.,.F.,.F.,(4,2,4),(-4.25163970020424,-2.12588055073164,
0.),.UNSPECIFIED.);
#148=B_SPLINE_CURVE_WITH_KNOTS('',3,(#12569,#12570,#12571,#12572,#12573,
#12574),.UNSPECIFIED.,.F.,.F.,(4,2,4),(-4.25163970020424,-2.1257591494726,
0.),.UNSPECIFIED.);
#201=CIRCLE('',#3254,7.5);
#202=CIRCLE('',#3255,1859.05088195134);
#203=CIRCLE('',#3257,7.5);
#204=CIRCLE('',#3258,1859.05088195135);
#205=CIRCLE('',#3264,25.);
#206=CIRCLE('',#3265,25.);
#362=FACE_OUTER_BOUND('',#554,.T.);
#363=FACE_OUTER_BOUND('',#555,.T.);
#364=FACE_OUTER_BOUND('',#556,.T.);
#365=FACE_OUTER_BOUND('',#557,.T.);
#366=FACE_OUTER_BOUND('',#558,.T.);
#367=FACE_OUTER_BOUND('',#559,.T.);
#368=FACE_OUTER_BOUND('',#560,.T.);
#369=FACE_OUTER_BOUND('',#561,.T.);
#370=FACE_OUTER_BOUND('',#562,.T.);
#371=FACE_OUTER_BOUND('',#563,.T.);
#372=FACE_OUTER_BOUND('',#564,.T.);
#373=FACE_OUTER_BOUND('',#565,.T.);
#374=FACE_OUTER_BOUND('',#566,.T.);
#375=FACE_OUTER_BOUND('',#567,.T.);
#376=FACE_OUTER_BOUND('',#569,.T.);
#554=EDGE_LOOP('',(#2597,#2598,#2599,#2600,#2601,#2602,#2603,#2604));
#555=EDGE_LOOP('',(#2605,#2606,#2607,#2608,#2609,#2610,#2611,#2612));
#556=EDGE_LOOP('',(#2613,#2614,#2615,#2616));
#557=EDGE_LOOP('',(#2617));
#558=EDGE_LOOP('',(#2618,#2619,#2620,#2621));
#559=EDGE_LOOP('',(#2622,#2623,#2624,#2625));
#560=EDGE_LOOP('',(#2626,#2627,#2628,#2629,#2630,#2631,#2632));
#561=EDGE_LOOP('',(#2633,#2634,#2635,#2636,#2637,#2638,#2639));
#562=EDGE_LOOP('',(#2640,#2641,#2642,#2643));
#563=EDGE_LOOP('',(#2644,#2645,#2646,#2647));
#564=EDGE_LOOP('',(#2648,#2649,#2650,#2651));
#565=EDGE_LOOP('',(#2652,#2653,#2654,#2655));
#566=EDGE_LOOP('',(#2656,#2657,#2658,#2659));
#567=EDGE_LOOP('',(#2660,#2661,#2662,#2663));
#568=EDGE_LOOP('',(#2664));
#569=EDGE_LOOP('',(#2665,#2666,#2667,#2668));
#774=(
BOUNDED_CURVE()
B_SPLINE_CURVE(2,(#11323,#11324,#11325,#11326,#11327,#11328,#11329,#11330,
#11331,#11332,#11333,#11334,#11335,#11336,#11337,#11338,#11339,#11340,#11341,
#11342,#11343,#11344,#11345,#11346,#11347,#11348,#11349,#11350,#11351,#11352,
#11353,#11354,#11355,#11356,#11357,#11358,#11359,#11360,#11361,#11362,#11363,
#11364,#11365),.UNSPECIFIED.,.F.,.F.)
B_SPLINE_CURVE_WITH_KNOTS((3,2,2,2,2,2,2,2,2,2,2,2,2,2,2,2,2,2,2,2,2,3),
(1.82334519084262E-6,0.0166666666666667,0.0333333333333333,0.05,0.0666666666666667,
0.0833333333333333,0.1,0.116666666666667,0.133333333333333,0.15,0.166666666666667,
0.183333333333333,0.2,0.216666666666667,0.233333333333333,0.25,0.266666666666667,
0.283333333333333,0.3,0.316666666666667,0.333333333333333,0.333335156678524),
 .UNSPECIFIED.)
CURVE()
GEOMETRIC_REPRESENTATION_ITEM()
RATIONAL_B_SPLINE_CURVE((0.999997306486108,0.987689687499436,1.,0.987688340595138,
1.,0.987688340595138,1.,0.987688340595138,1.,0.987688340595138,1.,0.987688340595138,
1.,0.987688340595138,1.,0.987688340595138,1.,0.987688340595138,1.,0.987688340595138,
1.,0.987688340595138,1.,0.987688340595138,1.,0.987688340595138,1.,0.987688340595138,
1.,0.987688340595138,1.,0.987688340595138,1.,0.987688340595138,1.,0.987688340595138,
1.,0.987688340595138,1.,0.987688340595138,1.,0.999998653095702,0.999997306486109))
REPRESENTATION_ITEM('')
);
#775=(
BOUNDED_CURVE()
B_SPLINE_CURVE(2,(#11370,#11371,#11372),.UNSPECIFIED.,.F.,.F.)
B_SPLINE_CURVE_WITH_KNOTS((3,3),(0.,1.82334519084262E-6),.UNSPECIFIED.)
CURVE()
GEOMETRIC_REPRESENTATION_ITEM()
RATIONAL_B_SPLINE_CURVE((1.,0.999998653095702,0.999997306486108))
REPRESENTATION_ITEM('')
);
#776=(
BOUNDED_CURVE()
B_SPLINE_CURVE(2,(#11746,#11747,#11748,#11749,#11750,#11751,#11752,#11753,
#11754,#11755,#11756,#11757,#11758,#11759,#11760,#11761,#11762,#11763,#11764,
#11765,#11766,#11767,#11768,#11769,#11770,#11771,#11772,#11773,#11774,#11775,
#11776,#11777,#11778,#11779,#11780,#11781,#11782,#11783,#11784,#11785,#11786),
 .UNSPECIFIED.,.F.,.F.)
B_SPLINE_CURVE_WITH_KNOTS((3,2,2,2,2,2,2,2,2,2,2,2,2,2,2,2,2,2,2,2,3),(0.666668490011857,
0.683333333333333,0.7,0.716666666666667,0.733333333333333,0.75,0.766666666666667,
0.783333333333333,0.8,0.816666666666667,0.833333333333333,0.85,0.866666666666667,
0.883333333333333,0.9,0.916666666666667,0.933333333333333,0.95,0.966666666666667,
0.983333333333333,1.),.UNSPECIFIED.)
CURVE()
GEOMETRIC_REPRESENTATION_ITEM()
RATIONAL_B_SPLINE_CURVE((0.999997306486109,0.987689687499436,1.,0.987688340595138,
1.,0.987688340595138,1.,0.987688340595138,1.,0.987688340595138,1.,0.987688340595138,
1.,0.987688340595138,1.,0.987688340595138,1.,0.987688340595138,1.,0.987688340595138,
1.,0.987688340595138,1.,0.987688340595138,1.,0.987688340595138,1.,0.987688340595138,
1.,0.987688340595138,1.,0.987688340595138,1.,0.987688340595138,1.,0.987688340595138,
1.,0.987688340595138,1.,0.987688340595138,1.))
REPRESENTATION_ITEM('')
);
#777=(
BOUNDED_CURVE()
B_SPLINE_CURVE(2,(#12151,#12152,#12153,#12154,#12155,#12156,#12157,#12158,
#12159,#12160,#12161,#12162,#12163,#12164,#12165,#12166,#12167,#12168,#12169,
#12170,#12171,#12172,#12173,#12174,#12175,#12176,#12177,#12178,#12179,#12180,
#12181,#12182,#12183,#12184,#12185,#12186,#12187,#12188,#12189,#12190,#12191,
#12192,#12193),.UNSPECIFIED.,.F.,.F.)
B_SPLINE_CURVE_WITH_KNOTS((3,2,2,2,2,2,2,2,2,2,2,2,2,2,2,2,2,2,2,2,2,3),
(0.333335156678524,0.35,0.366666666666667,0.383333333333333,0.4,0.416666666666667,
0.433333333333333,0.45,0.466666666666667,0.483333333333333,0.5,0.516666666666667,
0.533333333333333,0.55,0.566666666666667,0.583333333333333,0.6,0.616666666666667,
0.633333333333333,0.65,0.666666666666667,0.666668490011857),
 .UNSPECIFIED.)
CURVE()
GEOMETRIC_REPRESENTATION_ITEM()
RATIONAL_B_SPLINE_CURVE((0.999997306486109,0.987689687499436,1.,0.987688340595138,
1.,0.987688340595138,1.,0.987688340595138,1.,0.987688340595138,1.,0.987688340595138,
1.,0.987688340595138,1.,0.987688340595138,1.,0.987688340595138,1.,0.987688340595138,
1.,0.987688340595138,1.,0.987688340595138,1.,0.987688340595138,1.,0.987688340595138,
1.,0.987688340595138,1.,0.987688340595138,1.,0.987688340595138,1.,0.987688340595138,
1.,0.987688340595138,1.,0.987688340595138,1.,0.999998653095702,0.999997306486109))
REPRESENTATION_ITEM('')
);
#778=(
BOUNDED_CURVE()
B_SPLINE_CURVE(2,(#12820,#12821,#12822,#12823,#12824,#12825,#12826,#12827,
#12828,#12829,#12830,#12831,#12832,#12833,#12834,#12835,#12836,#12837,#12838,
#12839,#12840,#12841,#12842,#12843,#12844,#12845,#12846,#12847,#12848,#12849,
#12850,#12851,#12852,#12853,#12854,#12855,#12856,#12857,#12858,#12859,#12860,
#12861,#12862,#12863,#12864,#12865,#12866,#12867,#12868,#12869,#12870,#12871,
#12872,#12873,#12874,#12875,#12876,#12877,#12878,#12879,#12880,#12881,#12882,
#12883,#12884,#12885,#12886,#12887,#12888,#12889,#12890,#12891,#12892,#12893,
#12894,#12895,#12896,#12897,#12898,#12899,#12900,#12901,#12902,#12903,#12904,
#12905,#12906,#12907,#12908,#12909,#12910,#12911,#12912,#12913,#12914,#12915,
#12916,#12917,#12918,#12919,#12920,#12921,#12922,#12923,#12924,#12925,#12926,
#12927,#12928,#12929,#12930,#12931,#12932,#12933,#12934,#12935,#12936,#12937,
#12938,#12939,#12940),.UNSPECIFIED.,.F.,.F.)
B_SPLINE_CURVE_WITH_KNOTS((3,2,2,2,2,2,2,2,2,2,2,2,2,2,2,2,2,2,2,2,2,2,
2,2,2,2,2,2,2,2,2,2,2,2,2,2,2,2,2,2,2,2,2,2,2,2,2,2,2,2,2,2,2,2,2,2,2,2,
2,2,3),(0.,0.0166666666666667,0.0333333333333333,0.05,0.0666666666666667,
0.0833333333333333,0.1,0.116666666666667,0.133333333333333,0.15,0.166666666666667,
0.183333333333333,0.2,0.216666666666667,0.233333333333333,0.25,0.266666666666667,
0.283333333333333,0.3,0.316666666666667,0.333333333333333,0.35,0.366666666666667,
0.383333333333333,0.4,0.416666666666667,0.433333333333333,0.45,0.466666666666667,
0.483333333333333,0.5,0.516666666666667,0.533333333333333,0.55,0.566666666666667,
0.583333333333333,0.6,0.616666666666667,0.633333333333333,0.65,0.666666666666667,
0.683333333333333,0.7,0.716666666666667,0.733333333333333,0.75,0.766666666666667,
0.783333333333333,0.8,0.816666666666667,0.833333333333333,0.85,0.866666666666667,
0.883333333333333,0.9,0.916666666666667,0.933333333333333,0.95,0.966666666666667,
0.983333333333333,1.),.UNSPECIFIED.)
CURVE()
GEOMETRIC_REPRESENTATION_ITEM()
RATIONAL_B_SPLINE_CURVE((1.,0.987688340595138,1.,0.987688340595138,1.,0.987688340595138,
1.,0.987688340595138,1.,0.987688340595138,1.,0.987688340595138,1.,0.987688340595138,
1.,0.987688340595138,1.,0.987688340595138,1.,0.987688340595138,1.,0.987688340595138,
1.,0.987688340595138,1.,0.987688340595138,1.,0.987688340595138,1.,0.987688340595138,
1.,0.987688340595138,1.,0.987688340595138,1.,0.987688340595138,1.,0.987688340595138,
1.,0.987688340595138,1.,0.987688340595138,1.,0.987688340595138,1.,0.987688340595138,
1.,0.987688340595138,1.,0.987688340595138,1.,0.987688340595138,1.,0.987688340595138,
1.,0.987688340595138,1.,0.987688340595138,1.,0.987688340595138,1.,0.987688340595138,
1.,0.987688340595138,1.,0.987688340595138,1.,0.987688340595138,1.,0.987688340595138,
1.,0.987688340595138,1.,0.987688340595138,1.,0.987688340595138,1.,0.987688340595138,
1.,0.987688340595138,1.,0.987688340595138,1.,0.987688340595138,1.,0.987688340595138,
1.,0.987688340595138,1.,0.987688340595138,1.,0.987688340595138,1.,0.987688340595138,
1.,0.987688340595138,1.,0.987688340595138,1.,0.987688340595138,1.,0.987688340595138,
1.,0.987688340595138,1.,0.987688340595138,1.,0.987688340595138,1.,0.987688340595138,
1.,0.987688340595138,1.,0.987688340595138,1.,0.987688340595138,1.,0.987688340595138,
1.,0.987688340595138,1.))
REPRESENTATION_ITEM('')
);
#779=(
BOUNDED_CURVE()
B_SPLINE_CURVE(2,(#13183,#13184,#13185,#13186,#13187,#13188,#13189,#13190,
#13191,#13192,#13193,#13194,#13195,#13196,#13197,#13198,#13199,#13200,#13201,
#13202,#13203,#13204,#13205,#13206,#13207,#13208,#13209,#13210,#13211,#13212,
#13213,#13214,#13215,#13216,#13217,#13218,#13219,#13220,#13221,#13222,#13223,
#13224,#13225,#13226,#13227,#13228,#13229,#13230,#13231,#13232,#13233,#13234,
#13235,#13236,#13237,#13238,#13239,#13240,#13241,#13242,#13243,#13244,#13245,
#13246,#13247,#13248,#13249,#13250,#13251,#13252,#13253,#13254,#13255,#13256,
#13257,#13258,#13259,#13260,#13261,#13262,#13263,#13264,#13265,#13266,#13267,
#13268,#13269,#13270,#13271,#13272,#13273,#13274,#13275,#13276,#13277,#13278,
#13279,#13280,#13281,#13282,#13283,#13284,#13285,#13286,#13287,#13288,#13289,
#13290,#13291,#13292,#13293,#13294,#13295,#13296,#13297,#13298,#13299,#13300,
#13301,#13302,#13303),.UNSPECIFIED.,.F.,.F.)
B_SPLINE_CURVE_WITH_KNOTS((3,2,2,2,2,2,2,2,2,2,2,2,2,2,2,2,2,2,2,2,2,2,
2,2,2,2,2,2,2,2,2,2,2,2,2,2,2,2,2,2,2,2,2,2,2,2,2,2,2,2,2,2,2,2,2,2,2,2,
2,2,3),(0.,0.0166666666666667,0.0333333333333333,0.05,0.0666666666666667,
0.0833333333333333,0.1,0.116666666666667,0.133333333333333,0.15,0.166666666666667,
0.183333333333333,0.2,0.216666666666667,0.233333333333333,0.25,0.266666666666667,
0.283333333333333,0.3,0.316666666666667,0.333333333333333,0.35,0.366666666666667,
0.383333333333333,0.4,0.416666666666667,0.433333333333333,0.45,0.466666666666667,
0.483333333333333,0.5,0.516666666666667,0.533333333333333,0.55,0.566666666666667,
0.583333333333333,0.6,0.616666666666667,0.633333333333333,0.65,0.666666666666667,
0.683333333333333,0.7,0.716666666666667,0.733333333333333,0.75,0.766666666666667,
0.783333333333333,0.8,0.816666666666667,0.833333333333333,0.85,0.866666666666667,
0.883333333333333,0.9,0.916666666666667,0.933333333333333,0.95,0.966666666666667,
0.983333333333333,1.),.UNSPECIFIED.)
CURVE()
GEOMETRIC_REPRESENTATION_ITEM()
RATIONAL_B_SPLINE_CURVE((1.,0.987688340595138,1.,0.987688340595138,1.,0.987688340595138,
1.,0.987688340595138,1.,0.987688340595138,1.,0.987688340595138,1.,0.987688340595138,
1.,0.987688340595138,1.,0.987688340595138,1.,0.987688340595138,1.,0.987688340595138,
1.,0.987688340595138,1.,0.987688340595138,1.,0.987688340595138,1.,0.987688340595138,
1.,0.987688340595138,1.,0.987688340595138,1.,0.987688340595138,1.,0.987688340595138,
1.,0.987688340595138,1.,0.987688340595138,1.,0.987688340595138,1.,0.987688340595138,
1.,0.987688340595138,1.,0.987688340595138,1.,0.987688340595138,1.,0.987688340595138,
1.,0.987688340595138,1.,0.987688340595138,1.,0.987688340595138,1.,0.987688340595138,
1.,0.987688340595138,1.,0.987688340595138,1.,0.987688340595138,1.,0.987688340595138,
1.,0.987688340595138,1.,0.987688340595138,1.,0.987688340595138,1.,0.987688340595138,
1.,0.987688340595138,1.,0.987688340595138,1.,0.987688340595138,1.,0.987688340595138,
1.,0.987688340595138,1.,0.987688340595138,1.,0.987688340595138,1.,0.987688340595138,
1.,0.987688340595138,1.,0.987688340595138,1.,0.987688340595138,1.,0.987688340595138,
1.,0.987688340595138,1.,0.987688340595138,1.,0.987688340595138,1.,0.987688340595138,
1.,0.987688340595138,1.,0.987688340595138,1.,0.987688340595138,1.,0.987688340595138,
1.,0.987688340595138,1.))
REPRESENTATION_ITEM('')
);
#913=LINE('',#11321,#1064);
#914=LINE('',#11367,#1065);
#915=LINE('',#11383,#1066);
#916=LINE('',#11788,#1067);
#917=LINE('',#12565,#1068);
#918=LINE('',#12566,#1069);
#919=LINE('',#12576,#1070);
#920=LINE('',#12577,#1071);
#921=LINE('',#13551,#1072);
#922=LINE('',#13554,#1073);
#923=LINE('',#13557,#1074);
#924=LINE('',#13559,#1075);
#925=LINE('',#13560,#1076);
#926=LINE('',#13563,#1077);
#927=LINE('',#13565,#1078);
#928=LINE('',#13566,#1079);
#929=LINE('',#13568,#1080);
#930=LINE('',#13569,#1081);
#1064=VECTOR('',#3843,7.5);
#1065=VECTOR('',#3844,7.5);
#1066=VECTOR('',#3853,7.5);
#1067=VECTOR('',#3856,7.5);
#1068=VECTOR('',#3863,42.5163970020424);
#1069=VECTOR('',#3864,3.);
#1070=VECTOR('',#3867,3.);
#1071=VECTOR('',#3868,42.5163970020424);
#1072=VECTOR('',#3873,50.);
#1073=VECTOR('',#3876,50.);
#1074=VECTOR('',#3879,8.50510257216822);
#1075=VECTOR('',#3880,50.);
#1076=VECTOR('',#3881,8.50510257216822);
#1077=VECTOR('',#3884,10.);
#1078=VECTOR('',#3885,50.);
#1079=VECTOR('',#3886,10.);
#1080=VECTOR('',#3889,8.50510257216822);
#1081=VECTOR('',#3890,8.50510257216822);
#1346=VERTEX_POINT('',#11319);
#1347=VERTEX_POINT('',#11320);
#1348=VERTEX_POINT('',#11322);
#1349=VERTEX_POINT('',#11366);
#1350=VERTEX_POINT('',#11369);
#1351=VERTEX_POINT('',#11373);
#1352=VERTEX_POINT('',#11380);
#1353=VERTEX_POINT('',#11382);
#1354=VERTEX_POINT('',#11384);
#1355=VERTEX_POINT('',#11743);
#1356=VERTEX_POINT('',#11745);
#1357=VERTEX_POINT('',#11787);
#1358=VERTEX_POINT('',#12557);
#1359=VERTEX_POINT('',#12564);
#1360=VERTEX_POINT('',#12568);
#1361=VERTEX_POINT('',#12575);
#1362=VERTEX_POINT('',#13547);
#1363=VERTEX_POINT('',#13548);
#1364=VERTEX_POINT('',#13550);
#1365=VERTEX_POINT('',#13552);
#1366=VERTEX_POINT('',#13556);
#1367=VERTEX_POINT('',#13558);
#1368=VERTEX_POINT('',#13562);
#1369=VERTEX_POINT('',#13564);
#1767=EDGE_CURVE('',#1346,#1347,#913,.T.);
#1768=EDGE_CURVE('',#1348,#1346,#774,.T.);
#1769=EDGE_CURVE('',#1348,#1349,#914,.T.);
#1770=EDGE_CURVE('',#1349,#1349,#201,.T.);
#1771=EDGE_CURVE('',#1350,#1348,#775,.T.);
#1772=EDGE_CURVE('',#1350,#1351,#202,.T.);
#1773=EDGE_CURVE('',#1351,#1347,#143,.T.);
#1774=EDGE_CURVE('',#1352,#1352,#203,.T.);
#1775=EDGE_CURVE('',#1352,#1353,#915,.T.);
#1776=EDGE_CURVE('',#1353,#1354,#144,.T.);
#1777=EDGE_CURVE('',#1354,#1355,#204,.T.);
#1778=EDGE_CURVE('',#1356,#1355,#776,.T.);
#1779=EDGE_CURVE('',#1356,#1357,#916,.T.);
#1780=EDGE_CURVE('',#1357,#1353,#145,.T.);
#1781=EDGE_CURVE('',#1346,#1356,#777,.T.);
#1782=EDGE_CURVE('',#1347,#1357,#146,.T.);
#1783=EDGE_CURVE('',#1351,#1358,#147,.T.);
#1784=EDGE_CURVE('',#1359,#1350,#917,.T.);
#1785=EDGE_CURVE('',#1358,#1359,#918,.T.);
#1786=EDGE_CURVE('',#1360,#1354,#148,.T.);
#1787=EDGE_CURVE('',#1361,#1360,#919,.T.);
#1788=EDGE_CURVE('',#1355,#1361,#920,.T.);
#1789=EDGE_CURVE('',#1358,#1360,#778,.T.);
#1790=EDGE_CURVE('',#1359,#1361,#779,.T.);
#1791=EDGE_CURVE('',#1362,#1363,#205,.T.);
#1792=EDGE_CURVE('',#1364,#1363,#921,.T.);
#1793=EDGE_CURVE('',#1365,#1364,#206,.T.);
#1794=EDGE_CURVE('',#1365,#1362,#922,.T.);
#1795=EDGE_CURVE('',#1363,#1366,#923,.T.);
#1796=EDGE_CURVE('',#1367,#1366,#924,.T.);
#1797=EDGE_CURVE('',#1364,#1367,#925,.T.);
#1798=EDGE_CURVE('',#1366,#1368,#926,.T.);
#1799=EDGE_CURVE('',#1369,#1368,#927,.T.);
#1800=EDGE_CURVE('',#1367,#1369,#928,.T.);
#1801=EDGE_CURVE('',#1368,#1362,#929,.T.);
#1802=EDGE_CURVE('',#1369,#1365,#930,.T.);
#2597=ORIENTED_EDGE('',*,*,#1767,.F.);
#2598=ORIENTED_EDGE('',*,*,#1768,.F.);
#2599=ORIENTED_EDGE('',*,*,#1769,.T.);
#2600=ORIENTED_EDGE('',*,*,#1770,.F.);
#2601=ORIENTED_EDGE('',*,*,#1769,.F.);
#2602=ORIENTED_EDGE('',*,*,#1771,.F.);
#2603=ORIENTED_EDGE('',*,*,#1772,.T.);
#2604=ORIENTED_EDGE('',*,*,#1773,.T.);
#2605=ORIENTED_EDGE('',*,*,#1774,.T.);
#2606=ORIENTED_EDGE('',*,*,#1775,.T.);
#2607=ORIENTED_EDGE('',*,*,#1776,.T.);
#2608=ORIENTED_EDGE('',*,*,#1777,.T.);
#2609=ORIENTED_EDGE('',*,*,#1778,.F.);
#2610=ORIENTED_EDGE('',*,*,#1779,.T.);
#2611=ORIENTED_EDGE('',*,*,#1780,.T.);
#2612=ORIENTED_EDGE('',*,*,#1775,.F.);
#2613=ORIENTED_EDGE('',*,*,#1779,.F.);
#2614=ORIENTED_EDGE('',*,*,#1781,.F.);
#2615=ORIENTED_EDGE('',*,*,#1767,.T.);
#2616=ORIENTED_EDGE('',*,*,#1782,.T.);
#2617=ORIENTED_EDGE('',*,*,#1770,.T.);
#2618=ORIENTED_EDGE('',*,*,#1783,.F.);
#2619=ORIENTED_EDGE('',*,*,#1772,.F.);
#2620=ORIENTED_EDGE('',*,*,#1784,.F.);
#2621=ORIENTED_EDGE('',*,*,#1785,.F.);
#2622=ORIENTED_EDGE('',*,*,#1786,.F.);
#2623=ORIENTED_EDGE('',*,*,#1787,.F.);
#2624=ORIENTED_EDGE('',*,*,#1788,.F.);
#2625=ORIENTED_EDGE('',*,*,#1777,.F.);
#2626=ORIENTED_EDGE('',*,*,#1783,.T.);
#2627=ORIENTED_EDGE('',*,*,#1789,.T.);
#2628=ORIENTED_EDGE('',*,*,#1786,.T.);
#2629=ORIENTED_EDGE('',*,*,#1776,.F.);
#2630=ORIENTED_EDGE('',*,*,#1780,.F.);
#2631=ORIENTED_EDGE('',*,*,#1782,.F.);
#2632=ORIENTED_EDGE('',*,*,#1773,.F.);
#2633=ORIENTED_EDGE('',*,*,#1784,.T.);
#2634=ORIENTED_EDGE('',*,*,#1771,.T.);
#2635=ORIENTED_EDGE('',*,*,#1768,.T.);
#2636=ORIENTED_EDGE('',*,*,#1781,.T.);
#2637=ORIENTED_EDGE('',*,*,#1778,.T.);
#2638=ORIENTED_EDGE('',*,*,#1788,.T.);
#2639=ORIENTED_EDGE('',*,*,#1790,.F.);
#2640=ORIENTED_EDGE('',*,*,#1785,.T.);
#2641=ORIENTED_EDGE('',*,*,#1790,.T.);
#2642=ORIENTED_EDGE('',*,*,#1787,.T.);
#2643=ORIENTED_EDGE('',*,*,#1789,.F.);
#2644=ORIENTED_EDGE('',*,*,#1791,.T.);
#2645=ORIENTED_EDGE('',*,*,#1792,.F.);
#2646=ORIENTED_EDGE('',*,*,#1793,.F.);
#2647=ORIENTED_EDGE('',*,*,#1794,.T.);
#2648=ORIENTED_EDGE('',*,*,#1795,.T.);
#2649=ORIENTED_EDGE('',*,*,#1796,.F.);
#2650=ORIENTED_EDGE('',*,*,#1797,.F.);
#2651=ORIENTED_EDGE('',*,*,#1792,.T.);
#2652=ORIENTED_EDGE('',*,*,#1798,.T.);
#2653=ORIENTED_EDGE('',*,*,#1799,.F.);
#2654=ORIENTED_EDGE('',*,*,#1800,.F.);
#2655=ORIENTED_EDGE('',*,*,#1796,.T.);
#2656=ORIENTED_EDGE('',*,*,#1801,.T.);
#2657=ORIENTED_EDGE('',*,*,#1794,.F.);
#2658=ORIENTED_EDGE('',*,*,#1802,.F.);
#2659=ORIENTED_EDGE('',*,*,#1799,.T.);
#2660=ORIENTED_EDGE('',*,*,#1793,.T.);
#2661=ORIENTED_EDGE('',*,*,#1797,.T.);
#2662=ORIENTED_EDGE('',*,*,#1800,.T.);
#2663=ORIENTED_EDGE('',*,*,#1802,.T.);
#2664=ORIENTED_EDGE('',*,*,#1774,.F.);
#2665=ORIENTED_EDGE('',*,*,#1791,.F.);
#2666=ORIENTED_EDGE('',*,*,#1801,.F.);
#2667=ORIENTED_EDGE('',*,*,#1798,.F.);
#2668=ORIENTED_EDGE('',*,*,#1795,.F.);
#2790=CYLINDRICAL_SURFACE('',#3253,7.5);
#2791=CYLINDRICAL_SURFACE('',#3256,7.5);
#2792=CYLINDRICAL_SURFACE('',#3259,7.5);
#2793=CYLINDRICAL_SURFACE('',#3263,25.);
#2949=ADVANCED_FACE('',(#362),#2790,.T.);
#2950=ADVANCED_FACE('',(#363),#2791,.T.);
#2951=ADVANCED_FACE('',(#364),#2792,.T.);
#2952=ADVANCED_FACE('',(#365),#104,.T.);
#2953=ADVANCED_FACE('',(#366),#105,.F.);
#2954=ADVANCED_FACE('',(#367),#106,.F.);
#2955=ADVANCED_FACE('',(#368),#71,.T.);
#2956=ADVANCED_FACE('',(#369),#72,.T.);
#2957=ADVANCED_FACE('',(#370),#73,.T.);
#2958=ADVANCED_FACE('',(#371),#2793,.T.);
#2959=ADVANCED_FACE('',(#372),#107,.F.);
#2960=ADVANCED_FACE('',(#373),#108,.F.);
#2961=ADVANCED_FACE('',(#374),#109,.F.);
#2962=ADVANCED_FACE('',(#375,#134),#110,.T.);
#2963=ADVANCED_FACE('',(#376),#111,.F.);
#2969=CLOSED_SHELL('',(#2949,#2950,#2951,#2952,#2953,#2954,#2955,#2956,
#2957,#2958,#2959,#2960,#2961,#2962,#2963));
#3252=AXIS2_PLACEMENT_3D('',#11317,#3839,#3840);
#3253=AXIS2_PLACEMENT_3D('',#11318,#3841,#3842);
#3254=AXIS2_PLACEMENT_3D('',#11368,#3845,#3846);
#3255=AXIS2_PLACEMENT_3D('',#11374,#3847,#3848);
#3256=AXIS2_PLACEMENT_3D('',#11379,#3849,#3850);
#3257=AXIS2_PLACEMENT_3D('',#11381,#3851,#3852);
#3258=AXIS2_PLACEMENT_3D('',#11744,#3854,#3855);
#3259=AXIS2_PLACEMENT_3D('',#12150,#3857,#3858);
#3260=AXIS2_PLACEMENT_3D('',#12555,#3859,#3860);
#3261=AXIS2_PLACEMENT_3D('',#12556,#3861,#3862);
#3262=AXIS2_PLACEMENT_3D('',#12567,#3865,#3866);
#3263=AXIS2_PLACEMENT_3D('',#13546,#3869,#3870);
#3264=AXIS2_PLACEMENT_3D('',#13549,#3871,#3872);
#3265=AXIS2_PLACEMENT_3D('',#13553,#3874,#3875);
#3266=AXIS2_PLACEMENT_3D('',#13555,#3877,#3878);
#3267=AXIS2_PLACEMENT_3D('',#13561,#3882,#3883);
#3268=AXIS2_PLACEMENT_3D('',#13567,#3887,#3888);
#3269=AXIS2_PLACEMENT_3D('',#13570,#3891,#3892);
#3270=AXIS2_PLACEMENT_3D('',#13571,#3893,#3894);
#3839=DIRECTION('axis',(0.,0.,1.));
#3840=DIRECTION('refdir',(1.,0.,0.));
#3841=DIRECTION('center_axis',(0.,-1.,0.));
#3842=DIRECTION('ref_axis',(0.,0.,-1.));
#3843=DIRECTION('',(0.,1.,0.));
#3844=DIRECTION('',(0.,1.,0.));
#3845=DIRECTION('center_axis',(0.,1.,0.));
#3846=DIRECTION('ref_axis',(0.,0.,1.));
#3847=DIRECTION('center_axis',(0.997979715186782,0.0635333619109602,1.57664132857237E-12));
#3848=DIRECTION('ref_axis',(0.000102666233862281,-0.00161267745569481,0.999998694364682));
#3849=DIRECTION('center_axis',(0.,-1.,0.));
#3850=DIRECTION('ref_axis',(0.,0.,-1.));
#3851=DIRECTION('center_axis',(0.,1.,0.));
#3852=DIRECTION('ref_axis',(0.,0.,1.));
#3853=DIRECTION('',(0.,1.,0.));
#3854=DIRECTION('center_axis',(-0.997979715186782,-0.0635333619109597,-1.60052983355074E-12));
#3855=DIRECTION('ref_axis',(1.40886995536597E-7,-2.21307290245903E-6,0.999999999997541));
#3856=DIRECTION('',(0.,1.,0.));
#3857=DIRECTION('center_axis',(0.,-1.,0.));
#3858=DIRECTION('ref_axis',(0.,0.,-1.));
#3859=DIRECTION('center_axis',(0.,1.,0.));
#3860=DIRECTION('ref_axis',(0.,0.,1.));
#3861=DIRECTION('center_axis',(-0.997979715186782,-0.0635333619109615,0.));
#3862=DIRECTION('ref_axis',(0.,0.,1.));
#3863=DIRECTION('',(7.77774425693207E-18,0.,-1.));
#3864=DIRECTION('',(-0.0635333619109615,0.997979715186782,0.));
#3865=DIRECTION('center_axis',(0.997979715186782,0.063533361910961,0.));
#3866=DIRECTION('ref_axis',(0.,0.,-1.));
#3867=DIRECTION('',(0.0635333619109615,-0.997979715186782,0.));
#3868=DIRECTION('',(-7.77774425693207E-18,0.,1.));
#3869=DIRECTION('center_axis',(0.,-1.,0.));
#3870=DIRECTION('ref_axis',(-3.21624529935327E-16,0.,1.));
#3871=DIRECTION('center_axis',(0.,1.,0.));
#3872=DIRECTION('ref_axis',(0.,0.,1.));
#3873=DIRECTION('',(0.,-1.,0.));
#3874=DIRECTION('center_axis',(0.,1.,0.));
#3875=DIRECTION('ref_axis',(0.,0.,1.));
#3876=DIRECTION('',(0.,-1.,0.));
#3877=DIRECTION('center_axis',(-1.,0.,-4.07925350989523E-16));
#3878=DIRECTION('ref_axis',(-4.07925350989523E-16,0.,1.));
#3879=DIRECTION('',(3.91608336949942E-16,0.,-1.));
#3880=DIRECTION('',(0.,-1.,0.));
#3881=DIRECTION('',(3.91608336949942E-16,0.,-1.));
#3882=DIRECTION('center_axis',(0.,0.,1.));
#3883=DIRECTION('ref_axis',(1.,0.,0.));
#3884=DIRECTION('',(-1.,0.,0.));
#3885=DIRECTION('',(0.,-1.,0.));
#3886=DIRECTION('',(-1.,0.,0.));
#3887=DIRECTION('center_axis',(1.,0.,-4.07925350989523E-16));
#3888=DIRECTION('ref_axis',(-4.07925350989523E-16,0.,-1.));
#3889=DIRECTION('',(3.91608336949942E-16,0.,1.));
#3890=DIRECTION('',(3.91608336949942E-16,0.,1.));
#3891=DIRECTION('center_axis',(0.,1.,0.));
#3892=DIRECTION('ref_axis',(0.,0.,1.));
#3893=DIRECTION('center_axis',(0.,1.,0.));
#3894=DIRECTION('ref_axis',(0.,0.,1.));
#11317=CARTESIAN_POINT('',(0.,0.,0.));
#11318=CARTESIAN_POINT('Origin',(0.,240.,0.));
#11319=CARTESIAN_POINT('',(-1.90241102001116E-16,217.99585953923,7.50000000439337));
#11320=CARTESIAN_POINT('',(-4.06843950140785E-7,234.921557632927,7.50242802810186));
#11321=CARTESIAN_POINT('',(-9.18485099360515E-16,240.,7.5));
#11322=CARTESIAN_POINT('',(-9.18479639923619E-16,237.99585953923,7.50000000439337));
#11323=CARTESIAN_POINT('Ctrl Pts',(-9.1847417994869E-16,237.99585953923,
7.50000000439337));
#11324=CARTESIAN_POINT('Ctrl Pts',(-1.18775172812193,237.495912211348,7.50000000439337));
#11325=CARTESIAN_POINT('Ctrl Pts',(-2.317383311169,236.995967593475,7.13300320026677));
#11326=CARTESIAN_POINT('Ctrl Pts',(-3.44714003087638,236.495967593475,6.76596574150984));
#11327=CARTESIAN_POINT('Ctrl Pts',(-4.40818170865423,235.995967593475,6.06777834873578));
#11328=CARTESIAN_POINT('Ctrl Pts',(-5.36922338643209,235.495967593475,5.36959095596173));
#11329=CARTESIAN_POINT('Ctrl Pts',(-6.06747656688843,234.995967593475,4.40859707573286));
#11330=CARTESIAN_POINT('Ctrl Pts',(-6.76572974734476,234.495967593475,3.447603195504));
#11331=CARTESIAN_POINT('Ctrl Pts',(-7.13284454416054,233.995967593475,2.31787160445521));
#11332=CARTESIAN_POINT('Ctrl Pts',(-7.49995934097631,233.495967593475,1.18814001340642));
#11333=CARTESIAN_POINT('Ctrl Pts',(-7.5,232.995967593475,0.000256710972401669));
#11334=CARTESIAN_POINT('Ctrl Pts',(-7.50004065902369,232.495967593475,-1.18762659146162));
#11335=CARTESIAN_POINT('Ctrl Pts',(-7.13300320026677,231.995967593475,-2.317383311169));
#11336=CARTESIAN_POINT('Ctrl Pts',(-6.76596574150984,231.495967593475,-3.44714003087638));
#11337=CARTESIAN_POINT('Ctrl Pts',(-6.06777834873578,230.995967593475,-4.40818170865423));
#11338=CARTESIAN_POINT('Ctrl Pts',(-5.36959095596173,230.495967593475,-5.36922338643209));
#11339=CARTESIAN_POINT('Ctrl Pts',(-4.40859707573286,229.995967593475,-6.06747656688843));
#11340=CARTESIAN_POINT('Ctrl Pts',(-3.447603195504,229.495967593475,-6.76572974734476));
#11341=CARTESIAN_POINT('Ctrl Pts',(-2.31787160445521,228.995967593475,-7.13284454416054));
#11342=CARTESIAN_POINT('Ctrl Pts',(-1.18814001340642,228.495967593475,-7.49995934097631));
#11343=CARTESIAN_POINT('Ctrl Pts',(-0.000256710972402128,227.995967593475,
-7.5));
#11344=CARTESIAN_POINT('Ctrl Pts',(1.18762659146162,227.495967593475,-7.50004065902369));
#11345=CARTESIAN_POINT('Ctrl Pts',(2.317383311169,226.995967593475,-7.13300320026677));
#11346=CARTESIAN_POINT('Ctrl Pts',(3.44714003087638,226.495967593475,-6.76596574150984));
#11347=CARTESIAN_POINT('Ctrl Pts',(4.40818170865423,225.995967593475,-6.06777834873578));
#11348=CARTESIAN_POINT('Ctrl Pts',(5.36922338643209,225.495967593475,-5.36959095596173));
#11349=CARTESIAN_POINT('Ctrl Pts',(6.06747656688843,224.995967593475,-4.40859707573286));
#11350=CARTESIAN_POINT('Ctrl Pts',(6.76572974734476,224.495967593475,-3.447603195504));
#11351=CARTESIAN_POINT('Ctrl Pts',(7.13284454416054,223.995967593475,-2.31787160445521));
#11352=CARTESIAN_POINT('Ctrl Pts',(7.49995934097631,223.495967593475,-1.18814001340642));
#11353=CARTESIAN_POINT('Ctrl Pts',(7.5,222.995967593475,-0.000256710972402588));
#11354=CARTESIAN_POINT('Ctrl Pts',(7.50004065902369,222.495967593475,1.18762659146162));
#11355=CARTESIAN_POINT('Ctrl Pts',(7.13300320026677,221.995967593475,2.317383311169));
#11356=CARTESIAN_POINT('Ctrl Pts',(6.76596574150984,221.495967593475,3.44714003087638));
#11357=CARTESIAN_POINT('Ctrl Pts',(6.06777834873579,220.995967593475,4.40818170865423));
#11358=CARTESIAN_POINT('Ctrl Pts',(5.36959095596173,220.495967593475,5.36922338643209));
#11359=CARTESIAN_POINT('Ctrl Pts',(4.40859707573286,219.995967593475,6.06747656688843));
#11360=CARTESIAN_POINT('Ctrl Pts',(3.447603195504,219.495967593475,6.76572974734476));
#11361=CARTESIAN_POINT('Ctrl Pts',(2.31787160445521,218.995967593475,7.13284454416054));
#11362=CARTESIAN_POINT('Ctrl Pts',(1.18814001340643,218.495967593475,7.49995934097631));
#11363=CARTESIAN_POINT('Ctrl Pts',(0.00025671097240121,217.995967593475,
7.5));
#11364=CARTESIAN_POINT('Ctrl Pts',(0.000128355486249734,217.995913566499,
7.50000000439337));
#11365=CARTESIAN_POINT('Ctrl Pts',(5.38002895896315E-16,217.99585953923,
7.50000000439337));
#11366=CARTESIAN_POINT('',(0.,240.,7.5));
#11367=CARTESIAN_POINT('',(-9.18485099360515E-16,240.,7.5));
#11368=CARTESIAN_POINT('Origin',(0.,240.,0.));
#11369=CARTESIAN_POINT('',(0.00025671099249169,237.995967593476,7.49999999788428));
#11370=CARTESIAN_POINT('Ctrl Pts',(0.00025671097240121,237.995967593475,
7.5));
#11371=CARTESIAN_POINT('Ctrl Pts',(0.000128355486236195,237.995913566499,
7.50000000439337));
#11372=CARTESIAN_POINT('Ctrl Pts',(-9.1847417994869E-16,237.99585953923,
7.50000000439337));
#11373=CARTESIAN_POINT('',(0.19085679599498,235.002028447937,7.49999995822451));
#11374=CARTESIAN_POINT('Origin',(-5.20522648770767E-6,238.000081810591,
-1851.55088195117));
#11375=CARTESIAN_POINT('Ctrl Pts',(0.190856796705285,235.002028447915,7.5));
#11376=CARTESIAN_POINT('Ctrl Pts',(0.127311648028415,234.975281229334,7.50161706980302));
#11377=CARTESIAN_POINT('Ctrl Pts',(0.0636823578853783,234.948453397593,
7.50242803155527));
#11378=CARTESIAN_POINT('Ctrl Pts',(-4.06843934450864E-7,234.921557632927,
7.50242802810186));
#11379=CARTESIAN_POINT('Origin',(0.,240.,0.));
#11380=CARTESIAN_POINT('',(0.,150.,7.5));
#11381=CARTESIAN_POINT('Origin',(0.,150.,0.));
#11382=CARTESIAN_POINT('',(-4.0684396522591E-7,194.921557632927,7.50242802810186));
#11383=CARTESIAN_POINT('',(-9.18485099360515E-16,240.,7.5));
#11384=CARTESIAN_POINT('',(0.190870214476193,175.002034095778,7.4999996458277));
#11385=CARTESIAN_POINT('Ctrl Pts',(-4.06843965232862E-7,194.921557632927,
7.50242802810186));
#11386=CARTESIAN_POINT('Ctrl Pts',(-0.152090385415712,194.857323985265,
7.50242801985428));
#11387=CARTESIAN_POINT('Ctrl Pts',(-0.304485788637936,194.792702491972,
7.49779895914529));
#11388=CARTESIAN_POINT('Ctrl Pts',(-0.456762644214526,194.727870534021,
7.48851081348613));
#11389=CARTESIAN_POINT('Ctrl Pts',(-0.609070650330248,194.663025313709,
7.47922076779598));
#11390=CARTESIAN_POINT('Ctrl Pts',(-0.761259533137463,194.597969762789,
7.46526968655078));
#11391=CARTESIAN_POINT('Ctrl Pts',(-0.91290272043789,194.532885263598,7.44667945730617));
#11392=CARTESIAN_POINT('Ctrl Pts',(-1.06450493068591,194.467818351553,7.42809425151703));
#11393=CARTESIAN_POINT('Ctrl Pts',(-1.2155612127976,194.402722732839,7.40487246128588));
#11394=CARTESIAN_POINT('Ctrl Pts',(-1.36565093134532,194.337780178401,7.37708776215684));
#11395=CARTESIAN_POINT('Ctrl Pts',(-1.51579830432436,194.272812677376,7.34929239000474));
#11396=CARTESIAN_POINT('Ctrl Pts',(-1.6649778616245,194.207998581557,7.31693074896081));
#11397=CARTESIAN_POINT('Ctrl Pts',(-1.81278187771196,194.143517028959,7.28012693438018));
#11398=CARTESIAN_POINT('Ctrl Pts',(-1.92135204017681,194.096151789321,7.25309251248746));
#11399=CARTESIAN_POINT('Ctrl Pts',(-2.02918025203168,194.04896593395,7.22366229239575));
#11400=CARTESIAN_POINT('Ctrl Pts',(-2.13611185762632,194.002028447915,7.19190186588755));
#11401=CARTESIAN_POINT('Ctrl Pts',(-2.2816613117044,193.938139708658,7.14867131011455));
#11402=CARTESIAN_POINT('Ctrl Pts',(-2.42624566734731,193.87379055128,7.10091475754277));
#11403=CARTESIAN_POINT('Ctrl Pts',(-2.56944875671864,193.809155844927,7.04871331545309));
#11404=CARTESIAN_POINT('Ctrl Pts',(-2.71813540129491,193.74204613624,6.99451296753858));
#11405=CARTESIAN_POINT('Ctrl Pts',(-2.86533230206808,193.674628800623,6.93552054364116));
#11406=CARTESIAN_POINT('Ctrl Pts',(-3.01058579312346,193.607105531561,6.87188471229631));
#11407=CARTESIAN_POINT('Ctrl Pts',(-3.15046347852857,193.542081286575,6.81060403165537));
#11408=CARTESIAN_POINT('Ctrl Pts',(-3.28853853492898,193.476959054234,6.74501779444794));
#11409=CARTESIAN_POINT('Ctrl Pts',(-3.42442461876489,193.411920847683,6.67530840839924));
#11410=CARTESIAN_POINT('Ctrl Pts',(-3.5602870648691,193.346893954694,6.60561114847646));
#11411=CARTESIAN_POINT('Ctrl Pts',(-3.693960843474,193.281951283189,6.53179244342482));
#11412=CARTESIAN_POINT('Ctrl Pts',(-3.82508551083643,193.217273190526,6.45407988420021));
#11413=CARTESIAN_POINT('Ctrl Pts',(-3.95624536474471,193.152577741872,6.37634647125995));
#11414=CARTESIAN_POINT('Ctrl Pts',(-4.0848543388159,193.088147231022,6.2947174573996));
#11415=CARTESIAN_POINT('Ctrl Pts',(-4.21058385833655,193.024157275819,6.20946132033724));
#11416=CARTESIAN_POINT('Ctrl Pts',(-4.22508868089454,193.016775056041,6.1996257213086));
#11417=CARTESIAN_POINT('Ctrl Pts',(-4.23955521930311,193.009398692253,6.18974188939153));
#11418=CARTESIAN_POINT('Ctrl Pts',(-4.25398300016701,193.002028447915,6.17981026821526));
#11419=CARTESIAN_POINT('Ctrl Pts',(-4.37904978050105,192.938139708658,6.09371831161215));
#11420=CARTESIAN_POINT('Ctrl Pts',(-4.50180008775214,192.87379055128,6.00362010807856));
#11421=CARTESIAN_POINT('Ctrl Pts',(-4.62186318631576,192.809155844927,5.90972139815641));
#11422=CARTESIAN_POINT('Ctrl Pts',(-4.74652375991947,192.74204613624,5.8122271040762));
#11423=CARTESIAN_POINT('Ctrl Pts',(-4.86828667005456,192.674628800622,5.71063563105828));
#11424=CARTESIAN_POINT('Ctrl Pts',(-4.98676639590067,192.607105531561,5.6052285617595));
#11425=CARTESIAN_POINT('Ctrl Pts',(-5.10086120834454,192.542081286575,5.50372258918893));
#11426=CARTESIAN_POINT('Ctrl Pts',(-5.21191112857775,192.476959054234,5.39867883198654));
#11427=CARTESIAN_POINT('Ctrl Pts',(-5.31960508912721,192.411920847683,5.29039015693365));
#11428=CARTESIAN_POINT('Ctrl Pts',(-5.42728031603782,192.346893954693,5.18212031897172));
#11429=CARTESIAN_POINT('Ctrl Pts',(-5.53160039987492,192.281951283188,5.07060708921572));
#11430=CARTESIAN_POINT('Ctrl Pts',(-5.632292867741,192.217273190525,4.95617830276943));
#11431=CARTESIAN_POINT('Ctrl Pts',(-5.73301235584602,192.152577741871,4.84171881002288));
#11432=CARTESIAN_POINT('Ctrl Pts',(-5.83010200617219,192.088147231023,4.72434264585674));
#11433=CARTESIAN_POINT('Ctrl Pts',(-5.92333228977468,192.02415727582,4.60440668292466));
#11434=CARTESIAN_POINT('Ctrl Pts',(-5.93408782853699,192.016775056042,4.59057023570531));
#11435=CARTESIAN_POINT('Ctrl Pts',(-5.94479205212731,192.009398692253,4.5766997467359));
#11436=CARTESIAN_POINT('Ctrl Pts',(-5.95544464740897,192.002028447915,4.56279578422008));
#11437=CARTESIAN_POINT('Ctrl Pts',(-6.04778634614874,191.938139708657,4.44226970733661));
#11438=CARTESIAN_POINT('Ctrl Pts',(-6.13668694968295,191.87379055128,4.31864929275364));
#11439=CARTESIAN_POINT('Ctrl Pts',(-6.22185744482296,191.809155844926,4.19224477495645));
#11440=CARTESIAN_POINT('Ctrl Pts',(-6.31028930194836,191.742046136239,4.0609999554979));
#11441=CARTESIAN_POINT('Ctrl Pts',(-6.39469921942917,191.674628800622,3.92675391456802));
#11442=CARTESIAN_POINT('Ctrl Pts',(-6.47480755900329,191.60710553156,3.78989358567263));
#11443=CARTESIAN_POINT('Ctrl Pts',(-6.55195110329862,191.542081286575,3.65809843300132));
#11444=CARTESIAN_POINT('Ctrl Pts',(-6.6251055474419,191.476959054234,3.5238795706418));
#11445=CARTESIAN_POINT('Ctrl Pts',(-6.69406554949839,191.411920847682,3.38761165659044));
#11446=CARTESIAN_POINT('Ctrl Pts',(-6.76301355578597,191.346893954693,3.2513674466916));
#11447=CARTESIAN_POINT('Ctrl Pts',(-6.82776836820671,191.281951283189,3.11307538412042));
#11448=CARTESIAN_POINT('Ctrl Pts',(-6.88817215625433,191.217273190527,2.97313145734446));
#11449=CARTESIAN_POINT('Ctrl Pts',(-6.94859215330858,191.152577741872,2.83314997742638));
#11450=CARTESIAN_POINT('Ctrl Pts',(-7.00465866845448,191.088147231024,2.69151625970926));
#11451=CARTESIAN_POINT('Ctrl Pts',(-7.05626368640816,191.024157275821,2.54864063860052));
#11452=CARTESIAN_POINT('Ctrl Pts',(-7.06221711430205,191.016775056042,2.53215775104821));
#11453=CARTESIAN_POINT('Ctrl Pts',(-7.06811121908795,191.009398692254,2.51565834512789));
#11454=CARTESIAN_POINT('Ctrl Pts',(-7.07394587853975,191.002028447915,2.49914305799789));
#11455=CARTESIAN_POINT('Ctrl Pts',(-7.12452344682944,190.938139708658,2.35598079299494));
#11456=CARTESIAN_POINT('Ctrl Pts',(-7.17087213616523,190.87379055128,2.21093899485705));
#11457=CARTESIAN_POINT('Ctrl Pts',(-7.21281294639898,190.809155844927,2.06440202409992));
#11458=CARTESIAN_POINT('Ctrl Pts',(-7.2563597607299,190.74204613624,1.91225383662786));
#11459=CARTESIAN_POINT('Ctrl Pts',(-7.29515405471514,190.674628800622,1.75849416561916));
#11460=CARTESIAN_POINT('Ctrl Pts',(-7.32904944559233,190.607105531561,1.60357741968119));
#11461=CARTESIAN_POINT('Ctrl Pts',(-7.36169037413291,190.542081286575,1.45439411472324));
#11462=CARTESIAN_POINT('Ctrl Pts',(-7.38978847549664,190.476959054234,1.30413842461194));
#11463=CARTESIAN_POINT('Ctrl Pts',(-7.41326423358634,190.411920847683,1.15323012442364));
#11464=CARTESIAN_POINT('Ctrl Pts',(-7.43673590800807,190.346893954693,1.00234807511892));
#11465=CARTESIAN_POINT('Ctrl Pts',(-7.45558679680081,190.281951283188,0.850814170351292));
#11466=CARTESIAN_POINT('Ctrl Pts',(-7.46978916139915,190.217273190524,0.69905378984192));
#11467=CARTESIAN_POINT('Ctrl Pts',(-7.48399533711969,190.15257774187,0.547252685314279));
#11468=CARTESIAN_POINT('Ctrl Pts',(-7.493550535944,190.088147231021,0.395225509155809));
#11469=CARTESIAN_POINT('Ctrl Pts',(-7.49847882953778,190.024157275818,0.243395891136868));
#11470=CARTESIAN_POINT('Ctrl Pts',(-7.49904738356042,190.01677505604,0.225880023131504));
#11471=CARTESIAN_POINT('Ctrl Pts',(-7.49955441349822,190.009398692253,0.208366777073135));
#11472=CARTESIAN_POINT('Ctrl Pts',(-7.5,190.002028447915,0.190856796705286));
#11473=CARTESIAN_POINT('Ctrl Pts',(-7.50386255306115,189.938139708658,0.0390720635508336));
#11474=CARTESIAN_POINT('Ctrl Pts',(-7.50312239555638,189.87379055128,-0.113193416375283));
#11475=CARTESIAN_POINT('Ctrl Pts',(-7.4977280621597,189.809155844927,-0.265518780412243));
#11476=CARTESIAN_POINT('Ctrl Pts',(-7.49212716810079,189.74204613624,-0.423677011229148));
#11477=CARTESIAN_POINT('Ctrl Pts',(-7.48150838279932,189.674628800622,-0.581899244411572));
#11478=CARTESIAN_POINT('Ctrl Pts',(-7.46587290795734,189.60710553156,-0.739708076931111));
#11479=CARTESIAN_POINT('Ctrl Pts',(-7.45081609923473,189.542081286575,-0.891676432865303));
#11480=CARTESIAN_POINT('Ctrl Pts',(-7.43110741988625,189.476959054234,-1.04326087688739));
#11481=CARTESIAN_POINT('Ctrl Pts',(-7.40680096324194,189.411920847682,-1.19403760735031));
#11482=CARTESIAN_POINT('Ctrl Pts',(-7.38249873476802,189.346893954693,-1.3447881098148));
#11483=CARTESIAN_POINT('Ctrl Pts',(-7.35360044359543,189.281951283189,-1.49473066237826));
#11484=CARTESIAN_POINT('Ctrl Pts',(-7.32021115834367,189.217273190526,-1.64345213319688));
#11485=CARTESIAN_POINT('Ctrl Pts',(-7.28681291327052,189.152577741871,-1.79221351256119));
#11486=CARTESIAN_POINT('Ctrl Pts',(-7.24892146633721,189.088147231023,-1.93975266792177));
#11487=CARTESIAN_POINT('Ctrl Pts',(-7.20669061985663,189.02415727582,-2.08567414197882));
#11488=CARTESIAN_POINT('Ctrl Pts',(-7.20181864597947,189.016775056041,-2.10250841524041));
#11489=CARTESIAN_POINT('Ctrl Pts',(-7.19688896944668,189.009398692253,-2.11932118289446));
#11490=CARTESIAN_POINT('Ctrl Pts',(-7.19190186588755,189.002028447915,-2.13611185762632));
#11491=CARTESIAN_POINT('Ctrl Pts',(-7.14867131011472,188.938139708658,-2.28166131170383));
#11492=CARTESIAN_POINT('Ctrl Pts',(-7.10091475754315,188.873790551281,-2.42624566734616));
#11493=CARTESIAN_POINT('Ctrl Pts',(-7.0487133154537,188.809155844928,-2.56944875671694));
#11494=CARTESIAN_POINT('Ctrl Pts',(-6.99451296753918,188.742046136241,-2.71813540129337));
#11495=CARTESIAN_POINT('Ctrl Pts',(-6.93552054364173,188.674628800623,-2.8653323020667));
#11496=CARTESIAN_POINT('Ctrl Pts',(-6.87188471229685,188.607105531561,-3.01058579312224));
#11497=CARTESIAN_POINT('Ctrl Pts',(-6.81060403165581,188.542081286576,-3.15046347852764));
#11498=CARTESIAN_POINT('Ctrl Pts',(-6.74501779444825,188.476959054235,-3.28853853492835));
#11499=CARTESIAN_POINT('Ctrl Pts',(-6.67530840839942,188.411920847683,-3.42442461876454));
#11500=CARTESIAN_POINT('Ctrl Pts',(-6.60561114847652,188.346893954694,-3.560287064869));
#11501=CARTESIAN_POINT('Ctrl Pts',(-6.53179244342476,188.281951283189,-3.69396084347412));
#11502=CARTESIAN_POINT('Ctrl Pts',(-6.4540798842,188.217273190526,-3.82508551083678));
#11503=CARTESIAN_POINT('Ctrl Pts',(-6.37634647125945,188.152577741871,-3.95624536474554));
#11504=CARTESIAN_POINT('Ctrl Pts',(-6.29471745739878,188.088147231022,-4.08485433881718));
#11505=CARTESIAN_POINT('Ctrl Pts',(-6.20946132033607,188.024157275818,-4.21058385833828));
#11506=CARTESIAN_POINT('Ctrl Pts',(-6.19962572130782,188.01677505604,-4.22508868089568));
#11507=CARTESIAN_POINT('Ctrl Pts',(-6.18974188939115,188.009398692253,-4.23955521930367));
#11508=CARTESIAN_POINT('Ctrl Pts',(-6.17981026821527,188.002028447915,-4.25398300016699));
#11509=CARTESIAN_POINT('Ctrl Pts',(-6.09371831161279,187.938139708658,-4.37904978050011));
#11510=CARTESIAN_POINT('Ctrl Pts',(-6.00362010807988,187.873790551281,-4.50180008775034));
#11511=CARTESIAN_POINT('Ctrl Pts',(-5.90972139815848,187.809155844928,-4.62186318631311));
#11512=CARTESIAN_POINT('Ctrl Pts',(-5.81222710407815,187.742046136241,-4.74652375991708));
#11513=CARTESIAN_POINT('Ctrl Pts',(-5.71063563106011,187.674628800624,-4.86828667005243));
#11514=CARTESIAN_POINT('Ctrl Pts',(-5.60522856176118,187.607105531562,-4.98676639589878));
#11515=CARTESIAN_POINT('Ctrl Pts',(-5.50372258919049,187.542081286576,-5.10086120834287));
#11516=CARTESIAN_POINT('Ctrl Pts',(-5.39867883198795,187.476959054235,-5.21191112857629));
#11517=CARTESIAN_POINT('Ctrl Pts',(-5.29039015693491,187.411920847684,-5.31960508912596));
#11518=CARTESIAN_POINT('Ctrl Pts',(-5.18212031897362,187.346893954694,-5.42728031603598));
#11519=CARTESIAN_POINT('Ctrl Pts',(-5.07060708921829,187.28195128319,-5.53160039987254));
#11520=CARTESIAN_POINT('Ctrl Pts',(-4.9561783027727,187.217273190527,-5.63229286773812));
#11521=CARTESIAN_POINT('Ctrl Pts',(-4.84171881002545,187.152577741872,-5.73301235584388));
#11522=CARTESIAN_POINT('Ctrl Pts',(-4.72434264585857,187.088147231023,-5.83010200617073));
#11523=CARTESIAN_POINT('Ctrl Pts',(-4.60440668292569,187.024157275821,-5.92333228977387));
#11524=CARTESIAN_POINT('Ctrl Pts',(-4.59057023570601,187.016775056042,-5.93408782853645));
#11525=CARTESIAN_POINT('Ctrl Pts',(-4.57669974673625,187.009398692254,-5.94479205212704));
#11526=CARTESIAN_POINT('Ctrl Pts',(-4.56279578422009,187.002028447915,-5.95544464740895));
#11527=CARTESIAN_POINT('Ctrl Pts',(-4.44226970733713,186.938139708658,-6.04778634614834));
#11528=CARTESIAN_POINT('Ctrl Pts',(-4.31864929275469,186.87379055128,-6.1366869496822));
#11529=CARTESIAN_POINT('Ctrl Pts',(-4.19224477495805,186.809155844927,-6.22185744482188));
#11530=CARTESIAN_POINT('Ctrl Pts',(-4.0609999554994,186.74204613624,-6.31028930194741));
#11531=CARTESIAN_POINT('Ctrl Pts',(-3.9267539145694,186.674628800622,-6.39469921942832));
#11532=CARTESIAN_POINT('Ctrl Pts',(-3.78989358567389,186.607105531561,-6.47480755900255));
#11533=CARTESIAN_POINT('Ctrl Pts',(-3.65809843300279,186.542081286575,-6.55195110329779));
#11534=CARTESIAN_POINT('Ctrl Pts',(-3.52387957064348,186.476959054235,-6.62510554744101));
#11535=CARTESIAN_POINT('Ctrl Pts',(-3.38761165659234,186.411920847683,-6.69406554949743));
#11536=CARTESIAN_POINT('Ctrl Pts',(-3.25136744669377,186.346893954695,-6.76301355578491));
#11537=CARTESIAN_POINT('Ctrl Pts',(-3.11307538412286,186.28195128319,-6.82776836820559));
#11538=CARTESIAN_POINT('Ctrl Pts',(-2.97313145734719,186.217273190528,-6.88817215625315));
#11539=CARTESIAN_POINT('Ctrl Pts',(-2.83314997742771,186.152577741873,-6.94859215330807));
#11540=CARTESIAN_POINT('Ctrl Pts',(-2.69151625970919,186.088147231024,-7.00465866845454));
#11541=CARTESIAN_POINT('Ctrl Pts',(-2.54864063859899,186.024157275821,-7.05626368640871));
#11542=CARTESIAN_POINT('Ctrl Pts',(-2.53215775104719,186.016775056042,-7.06221711430242));
#11543=CARTESIAN_POINT('Ctrl Pts',(-2.51565834512738,186.009398692254,-7.06811121908813));
#11544=CARTESIAN_POINT('Ctrl Pts',(-2.49914305799789,186.002028447915,-7.07394587853975));
#11545=CARTESIAN_POINT('Ctrl Pts',(-2.35598079299478,185.938139708658,-7.12452344682949));
#11546=CARTESIAN_POINT('Ctrl Pts',(-2.21093899485675,185.87379055128,-7.17087213616532));
#11547=CARTESIAN_POINT('Ctrl Pts',(-2.06440202409945,185.809155844927,-7.21281294639912));
#11548=CARTESIAN_POINT('Ctrl Pts',(-1.91225383662743,185.74204613624,-7.25635976073001));
#11549=CARTESIAN_POINT('Ctrl Pts',(-1.75849416561874,185.674628800622,-7.29515405471524));
#11550=CARTESIAN_POINT('Ctrl Pts',(-1.60357741968081,185.60710553156,-7.32904944559241));
#11551=CARTESIAN_POINT('Ctrl Pts',(-1.45439411472211,185.542081286575,-7.36169037413315));
#11552=CARTESIAN_POINT('Ctrl Pts',(-1.30413842461007,185.476959054234,-7.38978847549698));
#11553=CARTESIAN_POINT('Ctrl Pts',(-1.15323012442101,185.411920847682,-7.41326423358675));
#11554=CARTESIAN_POINT('Ctrl Pts',(-1.002348075116,185.346893954692,-7.43673590800846));
#11555=CARTESIAN_POINT('Ctrl Pts',(-0.850814170348105,185.281951283187,
-7.45558679680118));
#11556=CARTESIAN_POINT('Ctrl Pts',(-0.699053789838449,185.217273190523,
-7.46978916139948));
#11557=CARTESIAN_POINT('Ctrl Pts',(-0.547252685310788,185.152577741868,
-7.48399533711995));
#11558=CARTESIAN_POINT('Ctrl Pts',(-0.395225509152289,185.088147231019,
-7.49355053594419));
#11559=CARTESIAN_POINT('Ctrl Pts',(-0.243395891133334,185.024157275817,
-7.4984788295379));
#11560=CARTESIAN_POINT('Ctrl Pts',(-0.225880023129145,185.016775056039,
-7.49904738356049));
#11561=CARTESIAN_POINT('Ctrl Pts',(-0.208366777071962,185.009398692252,
-7.49955441349825));
#11562=CARTESIAN_POINT('Ctrl Pts',(-0.190856796705286,185.002028447915,
-7.5));
#11563=CARTESIAN_POINT('Ctrl Pts',(-0.0390720635516772,184.938139708658,
-7.50386255306113));
#11564=CARTESIAN_POINT('Ctrl Pts',(0.113193416373591,184.873790551281,-7.50312239555639));
#11565=CARTESIAN_POINT('Ctrl Pts',(0.265518780409704,184.809155844928,-7.49772806215979));
#11566=CARTESIAN_POINT('Ctrl Pts',(0.42367701122682,184.742046136241,-7.49212716810092));
#11567=CARTESIAN_POINT('Ctrl Pts',(0.581899244409438,184.674628800623,-7.48150838279949));
#11568=CARTESIAN_POINT('Ctrl Pts',(0.739708076929191,184.607105531561,-7.46587290795754));
#11569=CARTESIAN_POINT('Ctrl Pts',(0.891676432862843,184.542081286576,-7.45081609923501));
#11570=CARTESIAN_POINT('Ctrl Pts',(1.04326087688443,184.476959054235,-7.43110741988665));
#11571=CARTESIAN_POINT('Ctrl Pts',(1.19403760734682,184.411920847684,-7.4068009632425));
#11572=CARTESIAN_POINT('Ctrl Pts',(1.34478810981303,184.346893954694,-7.38249873476838));
#11573=CARTESIAN_POINT('Ctrl Pts',(1.49473066237817,184.281951283189,-7.35360044359548));
#11574=CARTESIAN_POINT('Ctrl Pts',(1.64345213319847,184.217273190525,-7.32021115834331));
#11575=CARTESIAN_POINT('Ctrl Pts',(1.79221351256205,184.152577741871,-7.28681291327029));
#11576=CARTESIAN_POINT('Ctrl Pts',(1.93975266792193,184.088147231022,-7.24892146633715));
#11577=CARTESIAN_POINT('Ctrl Pts',(2.08567414197828,184.02415727582,-7.20669061985679));
#11578=CARTESIAN_POINT('Ctrl Pts',(2.10250841524006,184.016775056042,-7.20181864597957));
#11579=CARTESIAN_POINT('Ctrl Pts',(2.11932118289428,184.009398692253,-7.19688896944673));
#11580=CARTESIAN_POINT('Ctrl Pts',(2.13611185762632,184.002028447915,-7.19190186588755));
#11581=CARTESIAN_POINT('Ctrl Pts',(2.28166131170458,183.938139708658,-7.14867131011449));
#11582=CARTESIAN_POINT('Ctrl Pts',(2.42624566734765,183.87379055128,-7.10091475754266));
#11583=CARTESIAN_POINT('Ctrl Pts',(2.56944875671915,183.809155844927,-7.0487133154529));
#11584=CARTESIAN_POINT('Ctrl Pts',(2.71813540129538,183.74204613624,-6.9945129675384));
#11585=CARTESIAN_POINT('Ctrl Pts',(2.86533230206852,183.674628800622,-6.93552054364098));
#11586=CARTESIAN_POINT('Ctrl Pts',(3.01058579312386,183.60710553156,-6.87188471229614));
#11587=CARTESIAN_POINT('Ctrl Pts',(3.15046347852959,183.542081286575,-6.81060403165491));
#11588=CARTESIAN_POINT('Ctrl Pts',(3.28853853493061,183.476959054234,-6.74501779444716));
#11589=CARTESIAN_POINT('Ctrl Pts',(3.4244246187671,183.411920847682,-6.6753084083981));
#11590=CARTESIAN_POINT('Ctrl Pts',(3.5602870648721,183.346893954692,-6.60561114847487));
#11591=CARTESIAN_POINT('Ctrl Pts',(3.69396084347772,183.281951283188,-6.53179244342274));
#11592=CARTESIAN_POINT('Ctrl Pts',(3.82508551084086,183.217273190524,-6.45407988419758));
#11593=CARTESIAN_POINT('Ctrl Pts',(3.95624536474775,183.15257774187,-6.37634647125802));
#11594=CARTESIAN_POINT('Ctrl Pts',(4.08485433881761,183.088147231021,-6.29471745739845));
#11595=CARTESIAN_POINT('Ctrl Pts',(4.21058385833698,183.024157275819,-6.20946132033695));
#11596=CARTESIAN_POINT('Ctrl Pts',(4.22508868089482,183.016775056041,-6.19962572130841));
#11597=CARTESIAN_POINT('Ctrl Pts',(4.23955521930325,183.009398692253,-6.18974188939143));
#11598=CARTESIAN_POINT('Ctrl Pts',(4.25398300016701,183.002028447915,-6.17981026821526));
#11599=CARTESIAN_POINT('Ctrl Pts',(4.37904978050103,182.938139708658,-6.09371831161216));
#11600=CARTESIAN_POINT('Ctrl Pts',(4.50180008775213,182.87379055128,-6.00362010807857));
#11601=CARTESIAN_POINT('Ctrl Pts',(4.62186318631574,182.809155844927,-5.90972139815642));
#11602=CARTESIAN_POINT('Ctrl Pts',(4.74652375991945,182.74204613624,-5.81222710407621));
#11603=CARTESIAN_POINT('Ctrl Pts',(4.86828667005454,182.674628800622,-5.7106356310583));
#11604=CARTESIAN_POINT('Ctrl Pts',(4.98676639590065,182.607105531561,-5.60522856175951));
#11605=CARTESIAN_POINT('Ctrl Pts',(5.10086120834469,182.542081286575,-5.5037225891888));
#11606=CARTESIAN_POINT('Ctrl Pts',(5.21191112857806,182.476959054234,-5.39867883198624));
#11607=CARTESIAN_POINT('Ctrl Pts',(5.31960508912767,182.411920847683,-5.29039015693319));
#11608=CARTESIAN_POINT('Ctrl Pts',(5.42728031603767,182.346893954693,-5.18212031897185));
#11609=CARTESIAN_POINT('Ctrl Pts',(5.53160039987421,182.281951283189,-5.07060708921647));
#11610=CARTESIAN_POINT('Ctrl Pts',(5.63229286773977,182.217273190526,-4.95617830277083));
#11611=CARTESIAN_POINT('Ctrl Pts',(5.73301235584584,182.152577741871,-4.84171881002315));
#11612=CARTESIAN_POINT('Ctrl Pts',(5.83010200617298,182.088147231022,-4.72434264585582));
#11613=CARTESIAN_POINT('Ctrl Pts',(5.92333228977637,182.024157275819,-4.60440668292248));
#11614=CARTESIAN_POINT('Ctrl Pts',(5.9340878285381,182.016775056041,-4.59057023570386));
#11615=CARTESIAN_POINT('Ctrl Pts',(5.94479205212786,182.009398692253,-4.57669974673518));
#11616=CARTESIAN_POINT('Ctrl Pts',(5.95544464740895,182.002028447915,-4.56279578422009));
#11617=CARTESIAN_POINT('Ctrl Pts',(6.04778634614845,181.938139708658,-4.442269707337));
#11618=CARTESIAN_POINT('Ctrl Pts',(6.1366869496824,181.87379055128,-4.3186492927544));
#11619=CARTESIAN_POINT('Ctrl Pts',(6.22185744482218,181.809155844927,-4.19224477495761));
#11620=CARTESIAN_POINT('Ctrl Pts',(6.31028930194767,181.74204613624,-4.06099995549899));
#11621=CARTESIAN_POINT('Ctrl Pts',(6.39469921942856,181.674628800622,-3.92675391456902));
#11622=CARTESIAN_POINT('Ctrl Pts',(6.47480755900275,181.60710553156,-3.78989358567354));
#11623=CARTESIAN_POINT('Ctrl Pts',(6.5519511032983,181.542081286575,-3.65809843300192));
#11624=CARTESIAN_POINT('Ctrl Pts',(6.62510554744178,181.476959054234,-3.52387957064205));
#11625=CARTESIAN_POINT('Ctrl Pts',(6.69406554949843,181.411920847682,-3.38761165659035));
#11626=CARTESIAN_POINT('Ctrl Pts',(6.76301355578636,181.346893954693,-3.25136744669082));
#11627=CARTESIAN_POINT('Ctrl Pts',(6.8277683682074,181.281951283189,-3.11307538411894));
#11628=CARTESIAN_POINT('Ctrl Pts',(6.88817215625527,181.217273190526,-2.97313145734227));
#11629=CARTESIAN_POINT('Ctrl Pts',(6.94859215331014,181.152577741871,-2.83314997742263));
#11630=CARTESIAN_POINT('Ctrl Pts',(7.00465866845655,181.088147231021,-2.69151625970395));
#11631=CARTESIAN_POINT('Ctrl Pts',(7.05626368641066,181.024157275818,-2.54864063859361));
#11632=CARTESIAN_POINT('Ctrl Pts',(7.0622171143037,181.01677505604,-2.5321577510436));
#11633=CARTESIAN_POINT('Ctrl Pts',(7.06811121908876,181.009398692253,-2.51565834512559));
#11634=CARTESIAN_POINT('Ctrl Pts',(7.07394587853975,181.002028447915,-2.4991430579979));
#11635=CARTESIAN_POINT('Ctrl Pts',(7.12452344682943,180.938139708658,-2.35598079299495));
#11636=CARTESIAN_POINT('Ctrl Pts',(7.17087213616523,180.87379055128,-2.21093899485704));
#11637=CARTESIAN_POINT('Ctrl Pts',(7.21281294639899,180.809155844927,-2.0644020240999));
#11638=CARTESIAN_POINT('Ctrl Pts',(7.2563597607299,180.74204613624,-1.91225383662784));
#11639=CARTESIAN_POINT('Ctrl Pts',(7.29515405471515,180.674628800622,-1.75849416561912));
#11640=CARTESIAN_POINT('Ctrl Pts',(7.32904944559233,180.607105531561,-1.60357741968115));
#11641=CARTESIAN_POINT('Ctrl Pts',(7.36169037413299,180.542081286575,-1.45439411472287));
#11642=CARTESIAN_POINT('Ctrl Pts',(7.38978847549676,180.476959054234,-1.30413842461125));
#11643=CARTESIAN_POINT('Ctrl Pts',(7.4132642335865,180.411920847682,-1.15323012442261));
#11644=CARTESIAN_POINT('Ctrl Pts',(7.43673590800803,180.346893954693,-1.00234807511903));
#11645=CARTESIAN_POINT('Ctrl Pts',(7.45558679680064,180.281951283189,-0.850814170352573));
#11646=CARTESIAN_POINT('Ctrl Pts',(7.46978916139892,180.217273190526,-0.699053789844363));
#11647=CARTESIAN_POINT('Ctrl Pts',(7.48399533711951,180.152577741871,-0.547252685316772));
#11648=CARTESIAN_POINT('Ctrl Pts',(7.49355053594387,180.088147231022,-0.39522550915836));
#11649=CARTESIAN_POINT('Ctrl Pts',(7.4984788295377,180.024157275819,-0.243395891139465));
#11650=CARTESIAN_POINT('Ctrl Pts',(7.49904738356037,180.016775056041,-0.225880023133238));
#11651=CARTESIAN_POINT('Ctrl Pts',(7.49955441349819,180.009398692253,-0.208366777073998));
#11652=CARTESIAN_POINT('Ctrl Pts',(7.5,180.002028447915,-0.190856796705287));
#11653=CARTESIAN_POINT('Ctrl Pts',(7.50386255306115,179.938139708658,-0.0390720635508177));
#11654=CARTESIAN_POINT('Ctrl Pts',(7.50312239555638,179.87379055128,0.113193416375312));
#11655=CARTESIAN_POINT('Ctrl Pts',(7.49772806215969,179.809155844927,0.265518780412289));
#11656=CARTESIAN_POINT('Ctrl Pts',(7.49212716810078,179.74204613624,0.42367701122919));
#11657=CARTESIAN_POINT('Ctrl Pts',(7.48150838279932,179.674628800622,0.581899244411606));
#11658=CARTESIAN_POINT('Ctrl Pts',(7.46587290795734,179.60710553156,0.739708076931141));
#11659=CARTESIAN_POINT('Ctrl Pts',(7.45081609923473,179.542081286575,0.891676432865285));
#11660=CARTESIAN_POINT('Ctrl Pts',(7.43110741988625,179.476959054234,1.04326087688732));
#11661=CARTESIAN_POINT('Ctrl Pts',(7.40680096324196,179.411920847682,1.1940376073502));
#11662=CARTESIAN_POINT('Ctrl Pts',(7.38249873476815,179.346893954694,1.34478810981401));
#11663=CARTESIAN_POINT('Ctrl Pts',(7.35360044359571,179.281951283189,1.4947306623768));
#11664=CARTESIAN_POINT('Ctrl Pts',(7.32021115834415,179.217273190527,1.64345213319477));
#11665=CARTESIAN_POINT('Ctrl Pts',(7.28681291327109,179.152577741872,1.79221351255885));
#11666=CARTESIAN_POINT('Ctrl Pts',(7.24892146633789,179.088147231024,1.93975266791923));
#11667=CARTESIAN_POINT('Ctrl Pts',(7.20669061985743,179.024157275821,2.08567414197607));
#11668=CARTESIAN_POINT('Ctrl Pts',(7.20181864598001,179.016775056042,2.10250841523858));
#11669=CARTESIAN_POINT('Ctrl Pts',(7.19688896944695,179.009398692254,2.11932118289354));
#11670=CARTESIAN_POINT('Ctrl Pts',(7.19190186588755,179.002028447915,2.13611185762632));
#11671=CARTESIAN_POINT('Ctrl Pts',(7.14867131011455,178.938139708658,2.2816613117044));
#11672=CARTESIAN_POINT('Ctrl Pts',(7.10091475754278,178.87379055128,2.42624566734728));
#11673=CARTESIAN_POINT('Ctrl Pts',(7.0487133154531,178.809155844927,2.56944875671861));
#11674=CARTESIAN_POINT('Ctrl Pts',(6.99451296753859,178.74204613624,2.71813540129489));
#11675=CARTESIAN_POINT('Ctrl Pts',(6.93552054364116,178.674628800623,2.86533230206808));
#11676=CARTESIAN_POINT('Ctrl Pts',(6.87188471229631,178.607105531561,3.01058579312346));
#11677=CARTESIAN_POINT('Ctrl Pts',(6.81060403165535,178.542081286575,3.15046347852861));
#11678=CARTESIAN_POINT('Ctrl Pts',(6.7450177944479,178.476959054234,3.28853853492906));
#11679=CARTESIAN_POINT('Ctrl Pts',(6.67530840839917,178.411920847683,3.42442461876501));
#11680=CARTESIAN_POINT('Ctrl Pts',(6.60561114847623,178.346893954694,3.56028706486955));
#11681=CARTESIAN_POINT('Ctrl Pts',(6.53179244342441,178.281951283189,3.69396084347474));
#11682=CARTESIAN_POINT('Ctrl Pts',(6.4540798841996,178.217273190526,3.82508551083747));
#11683=CARTESIAN_POINT('Ctrl Pts',(6.37634647126001,178.152577741872,3.95624536474455));
#11684=CARTESIAN_POINT('Ctrl Pts',(6.29471745740041,178.088147231023,4.08485433881459));
#11685=CARTESIAN_POINT('Ctrl Pts',(6.20946132033887,178.02415727582,4.21058385833414));
#11686=CARTESIAN_POINT('Ctrl Pts',(6.1996257213097,178.016775056042,4.22508868089293));
#11687=CARTESIAN_POINT('Ctrl Pts',(6.18974188939208,178.009398692254,4.23955521930231));
#11688=CARTESIAN_POINT('Ctrl Pts',(6.17981026821526,178.002028447915,4.25398300016701));
#11689=CARTESIAN_POINT('Ctrl Pts',(6.09371831161207,177.938139708658,4.37904978050116));
#11690=CARTESIAN_POINT('Ctrl Pts',(6.0036201080784,177.87379055128,4.50180008775236));
#11691=CARTESIAN_POINT('Ctrl Pts',(5.90972139815616,177.809155844927,4.62186318631608));
#11692=CARTESIAN_POINT('Ctrl Pts',(5.81222710407596,177.74204613624,4.74652375991976));
#11693=CARTESIAN_POINT('Ctrl Pts',(5.71063563105806,177.674628800622,4.86828667005482));
#11694=CARTESIAN_POINT('Ctrl Pts',(5.6052285617593,177.60710553156,4.98676639590089));
#11695=CARTESIAN_POINT('Ctrl Pts',(5.5037225891889,177.542081286575,5.10086120834457));
#11696=CARTESIAN_POINT('Ctrl Pts',(5.39867883198667,177.476959054235,5.2119111285776));
#11697=CARTESIAN_POINT('Ctrl Pts',(5.29039015693398,177.411920847683,5.31960508912689));
#11698=CARTESIAN_POINT('Ctrl Pts',(5.18212031897253,177.346893954694,5.42728031603702));
#11699=CARTESIAN_POINT('Ctrl Pts',(5.07060708921705,177.281951283189,5.53160039987369));
#11700=CARTESIAN_POINT('Ctrl Pts',(4.95617830277129,177.217273190526,5.63229286773936));
#11701=CARTESIAN_POINT('Ctrl Pts',(4.84171881002452,177.152577741872,5.73301235584465));
#11702=CARTESIAN_POINT('Ctrl Pts',(4.72434264585812,177.088147231023,5.83010200617108));
#11703=CARTESIAN_POINT('Ctrl Pts',(4.60440668292578,177.024157275821,5.92333228977381));
#11704=CARTESIAN_POINT('Ctrl Pts',(4.59057023570606,177.016775056042,5.93408782853641));
#11705=CARTESIAN_POINT('Ctrl Pts',(4.57669974673629,177.009398692254,5.94479205212701));
#11706=CARTESIAN_POINT('Ctrl Pts',(4.56279578422009,177.002028447915,5.95544464740895));
#11707=CARTESIAN_POINT('Ctrl Pts',(4.44226970733713,176.938139708658,6.04778634614834));
#11708=CARTESIAN_POINT('Ctrl Pts',(4.31864929275468,176.87379055128,6.1366869496822));
#11709=CARTESIAN_POINT('Ctrl Pts',(4.19224477495804,176.809155844927,6.22185744482189));
#11710=CARTESIAN_POINT('Ctrl Pts',(4.06099995549939,176.74204613624,6.31028930194742));
#11711=CARTESIAN_POINT('Ctrl Pts',(3.92675391456939,176.674628800622,6.39469921942833));
#11712=CARTESIAN_POINT('Ctrl Pts',(3.78989358567388,176.607105531561,6.47480755900255));
#11713=CARTESIAN_POINT('Ctrl Pts',(3.65809843300261,176.542081286575,6.5519511032979));
#11714=CARTESIAN_POINT('Ctrl Pts',(3.52387957064311,176.476959054234,6.62510554744121));
#11715=CARTESIAN_POINT('Ctrl Pts',(3.38761165659179,176.411920847683,6.69406554949771));
#11716=CARTESIAN_POINT('Ctrl Pts',(3.25136744669221,176.346893954694,6.76301355578569));
#11717=CARTESIAN_POINT('Ctrl Pts',(3.11307538412028,176.281951283189,6.82776836820679));
#11718=CARTESIAN_POINT('Ctrl Pts',(2.97313145734355,176.217273190526,6.88817215625472));
#11719=CARTESIAN_POINT('Ctrl Pts',(2.83314997742486,176.152577741872,6.94859215330921));
#11720=CARTESIAN_POINT('Ctrl Pts',(2.69151625970714,176.088147231023,7.00465866845531));
#11721=CARTESIAN_POINT('Ctrl Pts',(2.54864063859777,176.02415727582,7.05626368640916));
#11722=CARTESIAN_POINT('Ctrl Pts',(2.53215775104638,176.016775056042,7.06221711430271));
#11723=CARTESIAN_POINT('Ctrl Pts',(2.51565834512697,176.009398692253,7.06811121908827));
#11724=CARTESIAN_POINT('Ctrl Pts',(2.49914305799789,176.002028447915,7.07394587853975));
#11725=CARTESIAN_POINT('Ctrl Pts',(2.35598079328146,175.938139708785,7.12452344672821));
#11726=CARTESIAN_POINT('Ctrl Pts',(2.21093899543762,175.873790551538,7.17087213597972));
#11727=CARTESIAN_POINT('Ctrl Pts',(2.06440202497974,175.809155845315,7.21281294614716));
#11728=CARTESIAN_POINT('Ctrl Pts',(1.91225491695072,175.742046612748,7.25635945154735));
#11729=CARTESIAN_POINT('Ctrl Pts',(1.75849634827299,175.674629757621,7.2951535041046));
#11730=CARTESIAN_POINT('Ctrl Pts',(1.60358071781314,175.607106969111,7.32904872396865));
#11731=CARTESIAN_POINT('Ctrl Pts',(1.4543974295954,175.542082725982,7.36168971919407));
#11732=CARTESIAN_POINT('Ctrl Pts',(1.30414175318146,175.476960494159,7.38978788807506));
#11733=CARTESIAN_POINT('Ctrl Pts',(1.15323346356763,175.411922286781,7.41326371413808));
#11734=CARTESIAN_POINT('Ctrl Pts',(1.0023514247394,175.346895392924,7.43673545653627));
#11735=CARTESIAN_POINT('Ctrl Pts',(0.850817527325577,175.281952719209,7.45558641375475));
#11736=CARTESIAN_POINT('Ctrl Pts',(0.699057151026253,175.217274623013,7.46978884684485));
#11737=CARTESIAN_POINT('Ctrl Pts',(0.547256052215635,175.152579171467,7.4839950909346));
#11738=CARTESIAN_POINT('Ctrl Pts',(0.395228878633319,175.088148656398,7.49355035828583));
#11739=CARTESIAN_POINT('Ctrl Pts',(0.243399260074249,175.024158695687,7.49847872018344));
#11740=CARTESIAN_POINT('Ctrl Pts',(0.225886742935279,175.016777887553,7.49904717331543));
#11741=CARTESIAN_POINT('Ctrl Pts',(0.208376846698734,175.009402933151,7.49955412589778));
#11742=CARTESIAN_POINT('Ctrl Pts',(0.190870214739035,175.002034095791,7.4999996585316));
#11743=CARTESIAN_POINT('',(0.000256710970817156,177.995967593475,7.49999999788466));
#11744=CARTESIAN_POINT('Origin',(-5.20512090547431E-6,178.000081808606,
-1851.55088195117));
#11745=CARTESIAN_POINT('',(-1.89809114034451E-16,197.99585953923,7.50000000439337));
#11746=CARTESIAN_POINT('Ctrl Pts',(5.38866871829646E-16,197.99585953923,
7.50000000439337));
#11747=CARTESIAN_POINT('Ctrl Pts',(-1.18775172812192,197.495912211348,7.50000000439337));
#11748=CARTESIAN_POINT('Ctrl Pts',(-2.317383311169,196.995967593475,7.13300320026677));
#11749=CARTESIAN_POINT('Ctrl Pts',(-3.44714003087638,196.495967593475,6.76596574150984));
#11750=CARTESIAN_POINT('Ctrl Pts',(-4.40818170865423,195.995967593475,6.06777834873578));
#11751=CARTESIAN_POINT('Ctrl Pts',(-5.36922338643209,195.495967593475,5.36959095596173));
#11752=CARTESIAN_POINT('Ctrl Pts',(-6.06747656688843,194.995967593475,4.40859707573286));
#11753=CARTESIAN_POINT('Ctrl Pts',(-6.76572974734476,194.495967593475,3.447603195504));
#11754=CARTESIAN_POINT('Ctrl Pts',(-7.13284454416054,193.995967593475,2.31787160445521));
#11755=CARTESIAN_POINT('Ctrl Pts',(-7.49995934097631,193.495967593475,1.18814001340642));
#11756=CARTESIAN_POINT('Ctrl Pts',(-7.5,192.995967593475,0.000256710972401669));
#11757=CARTESIAN_POINT('Ctrl Pts',(-7.50004065902369,192.495967593475,-1.18762659146162));
#11758=CARTESIAN_POINT('Ctrl Pts',(-7.13300320026677,191.995967593475,-2.317383311169));
#11759=CARTESIAN_POINT('Ctrl Pts',(-6.76596574150984,191.495967593475,-3.44714003087638));
#11760=CARTESIAN_POINT('Ctrl Pts',(-6.06777834873578,190.995967593475,-4.40818170865423));
#11761=CARTESIAN_POINT('Ctrl Pts',(-5.36959095596173,190.495967593475,-5.36922338643209));
#11762=CARTESIAN_POINT('Ctrl Pts',(-4.40859707573286,189.995967593475,-6.06747656688843));
#11763=CARTESIAN_POINT('Ctrl Pts',(-3.447603195504,189.495967593475,-6.76572974734476));
#11764=CARTESIAN_POINT('Ctrl Pts',(-2.31787160445521,188.995967593475,-7.13284454416054));
#11765=CARTESIAN_POINT('Ctrl Pts',(-1.18814001340642,188.495967593475,-7.49995934097631));
#11766=CARTESIAN_POINT('Ctrl Pts',(-0.000256710972402128,187.995967593475,
-7.5));
#11767=CARTESIAN_POINT('Ctrl Pts',(1.18762659146162,187.495967593475,-7.50004065902369));
#11768=CARTESIAN_POINT('Ctrl Pts',(2.317383311169,186.995967593475,-7.13300320026677));
#11769=CARTESIAN_POINT('Ctrl Pts',(3.44714003087638,186.495967593475,-6.76596574150984));
#11770=CARTESIAN_POINT('Ctrl Pts',(4.40818170865423,185.995967593475,-6.06777834873578));
#11771=CARTESIAN_POINT('Ctrl Pts',(5.36922338643209,185.495967593475,-5.36959095596173));
#11772=CARTESIAN_POINT('Ctrl Pts',(6.06747656688843,184.995967593475,-4.40859707573286));
#11773=CARTESIAN_POINT('Ctrl Pts',(6.76572974734476,184.495967593475,-3.447603195504));
#11774=CARTESIAN_POINT('Ctrl Pts',(7.13284454416054,183.995967593475,-2.31787160445521));
#11775=CARTESIAN_POINT('Ctrl Pts',(7.49995934097631,183.495967593475,-1.18814001340642));
#11776=CARTESIAN_POINT('Ctrl Pts',(7.5,182.995967593475,-0.000256710972402588));
#11777=CARTESIAN_POINT('Ctrl Pts',(7.50004065902369,182.495967593475,1.18762659146162));
#11778=CARTESIAN_POINT('Ctrl Pts',(7.13300320026677,181.995967593475,2.317383311169));
#11779=CARTESIAN_POINT('Ctrl Pts',(6.76596574150984,181.495967593475,3.44714003087638));
#11780=CARTESIAN_POINT('Ctrl Pts',(6.06777834873579,180.995967593475,4.40818170865423));
#11781=CARTESIAN_POINT('Ctrl Pts',(5.36959095596173,180.495967593475,5.36922338643209));
#11782=CARTESIAN_POINT('Ctrl Pts',(4.40859707573286,179.995967593475,6.06747656688843));
#11783=CARTESIAN_POINT('Ctrl Pts',(3.447603195504,179.495967593475,6.76572974734476));
#11784=CARTESIAN_POINT('Ctrl Pts',(2.31787160445521,178.995967593475,7.13284454416054));
#11785=CARTESIAN_POINT('Ctrl Pts',(1.18814001340643,178.495967593475,7.49995934097631));
#11786=CARTESIAN_POINT('Ctrl Pts',(0.00025671097240121,177.995967593475,
7.5));
#11787=CARTESIAN_POINT('',(-4.06843942354914E-7,214.921557632927,7.50242802810186));
#11788=CARTESIAN_POINT('',(-9.18485099360515E-16,240.,7.5));
#11789=CARTESIAN_POINT('Ctrl Pts',(-4.068439266928E-7,214.921557632927,
7.50242802810187));
#11790=CARTESIAN_POINT('Ctrl Pts',(-0.152090385416069,214.857323985265,
7.50242801985428));
#11791=CARTESIAN_POINT('Ctrl Pts',(-0.304485788638696,214.792702491972,
7.49779895914527));
#11792=CARTESIAN_POINT('Ctrl Pts',(-0.456762644215681,214.72787053402,7.48851081348606));
#11793=CARTESIAN_POINT('Ctrl Pts',(-0.609070650331504,214.663025313709,
7.47922076779588));
#11794=CARTESIAN_POINT('Ctrl Pts',(-0.761259533138804,214.597969762788,
7.46526968655064));
#11795=CARTESIAN_POINT('Ctrl Pts',(-0.91290272043933,214.532885263597,7.44667945730599));
#11796=CARTESIAN_POINT('Ctrl Pts',(-1.0645049306871,214.467818351553,7.42809425151685));
#11797=CARTESIAN_POINT('Ctrl Pts',(-1.21556121279854,214.402722732839,7.40487246128572));
#11798=CARTESIAN_POINT('Ctrl Pts',(-1.36565093134601,214.3377801784,7.37708776215671));
#11799=CARTESIAN_POINT('Ctrl Pts',(-1.51579830432504,214.272812677376,7.3492923900046));
#11800=CARTESIAN_POINT('Ctrl Pts',(-1.66497786162516,214.207998581557,7.31693074896066));
#11801=CARTESIAN_POINT('Ctrl Pts',(-1.8127818777126,214.143517028959,7.28012693438002));
#11802=CARTESIAN_POINT('Ctrl Pts',(-1.92135204017723,214.096151789321,7.25309251248735));
#11803=CARTESIAN_POINT('Ctrl Pts',(-2.02918025203189,214.04896593395,7.22366229239569));
#11804=CARTESIAN_POINT('Ctrl Pts',(-2.13611185762632,214.002028447915,7.19190186588755));
#11805=CARTESIAN_POINT('Ctrl Pts',(-2.28166131170438,213.938139708658,7.14867131011455));
#11806=CARTESIAN_POINT('Ctrl Pts',(-2.42624566734726,213.87379055128,7.10091475754279));
#11807=CARTESIAN_POINT('Ctrl Pts',(-2.56944875671857,213.809155844927,7.04871331545311));
#11808=CARTESIAN_POINT('Ctrl Pts',(-2.71813540129485,213.74204613624,6.99451296753861));
#11809=CARTESIAN_POINT('Ctrl Pts',(-2.86533230206802,213.674628800623,6.93552054364118));
#11810=CARTESIAN_POINT('Ctrl Pts',(-3.01058579312341,213.607105531561,6.87188471229634));
#11811=CARTESIAN_POINT('Ctrl Pts',(-3.15046347852853,213.542081286575,6.81060403165539));
#11812=CARTESIAN_POINT('Ctrl Pts',(-3.28853853492897,213.476959054234,6.74501779444794));
#11813=CARTESIAN_POINT('Ctrl Pts',(-3.4244246187649,213.411920847683,6.67530840839923));
#11814=CARTESIAN_POINT('Ctrl Pts',(-3.56028706486959,213.346893954694,6.60561114847621));
#11815=CARTESIAN_POINT('Ctrl Pts',(-3.69396084347493,213.281951283189,6.53179244342431));
#11816=CARTESIAN_POINT('Ctrl Pts',(-3.8250855108378,213.217273190526,6.4540798841994));
#11817=CARTESIAN_POINT('Ctrl Pts',(-3.95624536474509,213.152577741871,6.37634647125968));
#11818=CARTESIAN_POINT('Ctrl Pts',(-4.08485433881534,213.088147231023,6.29471745739993));
#11819=CARTESIAN_POINT('Ctrl Pts',(-4.21058385833508,213.02415727582,6.20946132033823));
#11820=CARTESIAN_POINT('Ctrl Pts',(-4.22508868089356,213.016775056042,6.19962572130926));
#11821=CARTESIAN_POINT('Ctrl Pts',(-4.23955521930262,213.009398692253,6.18974188939186));
#11822=CARTESIAN_POINT('Ctrl Pts',(-4.25398300016701,213.002028447915,6.17981026821525));
#11823=CARTESIAN_POINT('Ctrl Pts',(-4.37904978050102,212.938139708658,6.09371831161217));
#11824=CARTESIAN_POINT('Ctrl Pts',(-4.50180008775209,212.87379055128,6.00362010807859));
#11825=CARTESIAN_POINT('Ctrl Pts',(-4.62186318631568,212.809155844927,5.90972139815647));
#11826=CARTESIAN_POINT('Ctrl Pts',(-4.74652375991939,212.74204613624,5.81222710407626));
#11827=CARTESIAN_POINT('Ctrl Pts',(-4.86828667005449,212.674628800623,5.71063563105834));
#11828=CARTESIAN_POINT('Ctrl Pts',(-4.9867663959006,212.607105531561,5.60522856175955));
#11829=CARTESIAN_POINT('Ctrl Pts',(-5.10086120834463,212.542081286575,5.50372258918886));
#11830=CARTESIAN_POINT('Ctrl Pts',(-5.21191112857799,212.476959054234,5.39867883198632));
#11831=CARTESIAN_POINT('Ctrl Pts',(-5.31960508912758,212.411920847683,5.29039015693328));
#11832=CARTESIAN_POINT('Ctrl Pts',(-5.42728031603771,212.346893954693,5.18212031897182));
#11833=CARTESIAN_POINT('Ctrl Pts',(-5.53160039987437,212.281951283189,5.07060708921631));
#11834=CARTESIAN_POINT('Ctrl Pts',(-5.63229286774003,212.217273190525,4.95617830277053));
#11835=CARTESIAN_POINT('Ctrl Pts',(-5.73301235584579,212.152577741871,4.84171881002319));
#11836=CARTESIAN_POINT('Ctrl Pts',(-5.83010200617264,212.088147231022,4.72434264585622));
#11837=CARTESIAN_POINT('Ctrl Pts',(-5.92333228977576,212.02415727582,4.60440668292327));
#11838=CARTESIAN_POINT('Ctrl Pts',(-5.9340878285377,212.016775056041,4.59057023570439));
#11839=CARTESIAN_POINT('Ctrl Pts',(-5.94479205212766,212.009398692253,4.57669974673545));
#11840=CARTESIAN_POINT('Ctrl Pts',(-5.95544464740895,212.002028447915,4.5627957842201));
#11841=CARTESIAN_POINT('Ctrl Pts',(-6.04778634614838,211.938139708658,4.44226970733709));
#11842=CARTESIAN_POINT('Ctrl Pts',(-6.13668694968226,211.87379055128,4.3186492927546));
#11843=CARTESIAN_POINT('Ctrl Pts',(-6.22185744482198,211.809155844927,4.19224477495791));
#11844=CARTESIAN_POINT('Ctrl Pts',(-6.3102893019475,211.74204613624,4.06099995549926));
#11845=CARTESIAN_POINT('Ctrl Pts',(-6.39469921942841,211.674628800622,3.92675391456926));
#11846=CARTESIAN_POINT('Ctrl Pts',(-6.47480755900262,211.607105531561,3.78989358567376));
#11847=CARTESIAN_POINT('Ctrl Pts',(-6.55195110329808,211.542081286575,3.65809843300229));
#11848=CARTESIAN_POINT('Ctrl Pts',(-6.62510554744149,211.476959054234,3.52387957064258));
#11849=CARTESIAN_POINT('Ctrl Pts',(-6.69406554949808,211.411920847683,3.38761165659104));
#11850=CARTESIAN_POINT('Ctrl Pts',(-6.76301355578619,211.346893954693,3.25136744669118));
#11851=CARTESIAN_POINT('Ctrl Pts',(-6.8277683682074,211.281951283189,3.11307538411895));
#11852=CARTESIAN_POINT('Ctrl Pts',(-6.88817215625542,211.217273190525,2.97313145734192));
#11853=CARTESIAN_POINT('Ctrl Pts',(-6.94859215330986,211.152577741871,2.83314997742328));
#11854=CARTESIAN_POINT('Ctrl Pts',(-7.00465866845589,211.088147231022,2.69151625970561));
#11855=CARTESIAN_POINT('Ctrl Pts',(-7.05626368640969,211.02415727582,2.5486406385963));
#11856=CARTESIAN_POINT('Ctrl Pts',(-7.06221711430306,211.016775056041,2.53215775104539));
#11857=CARTESIAN_POINT('Ctrl Pts',(-7.06811121908845,211.009398692253,2.51565834512648));
#11858=CARTESIAN_POINT('Ctrl Pts',(-7.07394587853975,211.002028447915,2.49914305799789));
#11859=CARTESIAN_POINT('Ctrl Pts',(-7.12452344682943,210.938139708658,2.35598079299496));
#11860=CARTESIAN_POINT('Ctrl Pts',(-7.17087213616521,210.87379055128,2.2109389948571));
#11861=CARTESIAN_POINT('Ctrl Pts',(-7.21281294639896,210.809155844927,2.06440202409999));
#11862=CARTESIAN_POINT('Ctrl Pts',(-7.25635976072988,210.74204613624,1.91225383662793));
#11863=CARTESIAN_POINT('Ctrl Pts',(-7.29515405471512,210.674628800622,1.75849416561922));
#11864=CARTESIAN_POINT('Ctrl Pts',(-7.32904944559231,210.607105531561,1.60357741968125));
#11865=CARTESIAN_POINT('Ctrl Pts',(-7.3616903741329,210.542081286575,1.4543941147233));
#11866=CARTESIAN_POINT('Ctrl Pts',(-7.38978847549662,210.476959054234,1.30413842461201));
#11867=CARTESIAN_POINT('Ctrl Pts',(-7.41326423358633,210.411920847683,1.15323012442371));
#11868=CARTESIAN_POINT('Ctrl Pts',(-7.43673590800795,210.346893954693,1.00234807511964));
#11869=CARTESIAN_POINT('Ctrl Pts',(-7.45558679680064,210.281951283189,0.85081417035268));
#11870=CARTESIAN_POINT('Ctrl Pts',(-7.46978916139896,210.217273190525,0.699053789843961));
#11871=CARTESIAN_POINT('Ctrl Pts',(-7.48399533711949,210.152577741871,0.54725268531685));
#11872=CARTESIAN_POINT('Ctrl Pts',(-7.49355053594383,210.088147231022,0.395225509158903));
#11873=CARTESIAN_POINT('Ctrl Pts',(-7.49847882953766,210.02415727582,0.243395891140488));
#11874=CARTESIAN_POINT('Ctrl Pts',(-7.49904738356035,210.016775056041,0.225880023133914));
#11875=CARTESIAN_POINT('Ctrl Pts',(-7.49955441349819,210.009398692253,0.208366777074336));
#11876=CARTESIAN_POINT('Ctrl Pts',(-7.5,210.002028447915,0.190856796705278));
#11877=CARTESIAN_POINT('Ctrl Pts',(-7.50386255306115,209.938139708658,0.0390720635509829));
#11878=CARTESIAN_POINT('Ctrl Pts',(-7.50312239555638,209.87379055128,-0.11319341637498));
#11879=CARTESIAN_POINT('Ctrl Pts',(-7.49772806215971,209.809155844927,-0.265518780411782));
#11880=CARTESIAN_POINT('Ctrl Pts',(-7.49212716810081,209.74204613624,-0.423677011228724));
#11881=CARTESIAN_POINT('Ctrl Pts',(-7.48150838279936,209.674628800622,-0.581899244411169));
#11882=CARTESIAN_POINT('Ctrl Pts',(-7.46587290795738,209.607105531561,-0.739708076930746));
#11883=CARTESIAN_POINT('Ctrl Pts',(-7.4508160992348,209.542081286575,-0.891676432864672));
#11884=CARTESIAN_POINT('Ctrl Pts',(-7.43110741988636,209.476959054234,-1.04326087688651));
#11885=CARTESIAN_POINT('Ctrl Pts',(-7.40680096324212,209.411920847683,-1.19403760734917));
#11886=CARTESIAN_POINT('Ctrl Pts',(-7.38249873476809,209.346893954693,-1.34478810981454));
#11887=CARTESIAN_POINT('Ctrl Pts',(-7.35360044359533,209.281951283189,-1.49473066237887));
#11888=CARTESIAN_POINT('Ctrl Pts',(-7.32021115834334,209.217273190525,-1.64345213319835));
#11889=CARTESIAN_POINT('Ctrl Pts',(-7.28681291327022,209.152577741871,-1.79221351256238));
#11890=CARTESIAN_POINT('Ctrl Pts',(-7.24892146633696,209.088147231022,-1.93975266792269));
#11891=CARTESIAN_POINT('Ctrl Pts',(-7.20669061985644,209.02415727582,-2.08567414197946));
#11892=CARTESIAN_POINT('Ctrl Pts',(-7.20181864597934,209.016775056041,-2.10250841524085));
#11893=CARTESIAN_POINT('Ctrl Pts',(-7.19688896944662,209.009398692253,-2.11932118289467));
#11894=CARTESIAN_POINT('Ctrl Pts',(-7.19190186588755,209.002028447915,-2.13611185762632));
#11895=CARTESIAN_POINT('Ctrl Pts',(-7.14867131011455,208.938139708658,-2.28166131170439));
#11896=CARTESIAN_POINT('Ctrl Pts',(-7.10091475754278,208.87379055128,-2.42624566734729));
#11897=CARTESIAN_POINT('Ctrl Pts',(-7.0487133154531,208.809155844927,-2.56944875671861));
#11898=CARTESIAN_POINT('Ctrl Pts',(-6.99451296753859,208.74204613624,-2.71813540129489));
#11899=CARTESIAN_POINT('Ctrl Pts',(-6.93552054364117,208.674628800623,-2.86533230206806));
#11900=CARTESIAN_POINT('Ctrl Pts',(-6.87188471229632,208.607105531561,-3.01058579312345));
#11901=CARTESIAN_POINT('Ctrl Pts',(-6.8106040316553,208.542081286575,-3.15046347852873));
#11902=CARTESIAN_POINT('Ctrl Pts',(-6.74501779444778,208.476959054234,-3.28853853492931));
#11903=CARTESIAN_POINT('Ctrl Pts',(-6.67530840839898,208.411920847683,-3.42442461876539));
#11904=CARTESIAN_POINT('Ctrl Pts',(-6.60561114847592,208.346893954693,-3.56028706487013));
#11905=CARTESIAN_POINT('Ctrl Pts',(-6.53179244342397,208.281951283189,-3.69396084347553));
#11906=CARTESIAN_POINT('Ctrl Pts',(-6.45407988419901,208.217273190525,-3.82508551083845));
#11907=CARTESIAN_POINT('Ctrl Pts',(-6.37634647125933,208.152577741871,-3.95624536474565));
#11908=CARTESIAN_POINT('Ctrl Pts',(-6.29471745739962,208.088147231022,-4.08485433881581));
#11909=CARTESIAN_POINT('Ctrl Pts',(-6.20946132033797,208.02415727582,-4.21058385833547));
#11910=CARTESIAN_POINT('Ctrl Pts',(-6.19962572130909,208.016775056041,-4.22508868089382));
#11911=CARTESIAN_POINT('Ctrl Pts',(-6.18974188939178,208.009398692253,-4.23955521930275));
#11912=CARTESIAN_POINT('Ctrl Pts',(-6.17981026821526,208.002028447915,-4.253983000167));
#11913=CARTESIAN_POINT('Ctrl Pts',(-6.09371831161218,207.938139708658,-4.379049780501));
#11914=CARTESIAN_POINT('Ctrl Pts',(-6.00362010807862,207.87379055128,-4.50180008775205));
#11915=CARTESIAN_POINT('Ctrl Pts',(-5.90972139815651,207.809155844927,-4.62186318631563));
#11916=CARTESIAN_POINT('Ctrl Pts',(-5.81222710407629,207.74204613624,-4.74652375991935));
#11917=CARTESIAN_POINT('Ctrl Pts',(-5.71063563105837,207.674628800623,-4.86828667005446));
#11918=CARTESIAN_POINT('Ctrl Pts',(-5.60522856175958,207.607105531561,-4.98676639590057));
#11919=CARTESIAN_POINT('Ctrl Pts',(-5.50372258918887,207.542081286575,-5.10086120834461));
#11920=CARTESIAN_POINT('Ctrl Pts',(-5.39867883198632,207.476959054234,-5.21191112857799));
#11921=CARTESIAN_POINT('Ctrl Pts',(-5.29039015693326,207.411920847683,-5.3196050891276));
#11922=CARTESIAN_POINT('Ctrl Pts',(-5.18212031897177,207.346893954693,-5.42728031603775));
#11923=CARTESIAN_POINT('Ctrl Pts',(-5.07060708921622,207.281951283189,-5.53160039987444));
#11924=CARTESIAN_POINT('Ctrl Pts',(-4.95617830277041,207.217273190525,-5.63229286774013));
#11925=CARTESIAN_POINT('Ctrl Pts',(-4.8417188100227,207.152577741871,-5.73301235584621));
#11926=CARTESIAN_POINT('Ctrl Pts',(-4.72434264585535,207.088147231022,-5.83010200617336));
#11927=CARTESIAN_POINT('Ctrl Pts',(-4.60440668292199,207.024157275819,-5.92333228977675));
#11928=CARTESIAN_POINT('Ctrl Pts',(-4.59057023570353,207.016775056041,-5.93408782853836));
#11929=CARTESIAN_POINT('Ctrl Pts',(-4.57669974673502,207.009398692253,-5.94479205212799));
#11930=CARTESIAN_POINT('Ctrl Pts',(-4.56279578422009,207.002028447915,-5.95544464740895));
#11931=CARTESIAN_POINT('Ctrl Pts',(-4.44226970733713,206.938139708658,-6.04778634614835));
#11932=CARTESIAN_POINT('Ctrl Pts',(-4.31864929275468,206.87379055128,-6.1366869496822));
#11933=CARTESIAN_POINT('Ctrl Pts',(-4.19224477495804,206.809155844927,-6.22185744482189));
#11934=CARTESIAN_POINT('Ctrl Pts',(-4.06099995549939,206.74204613624,-6.31028930194741));
#11935=CARTESIAN_POINT('Ctrl Pts',(-3.92675391456938,206.674628800622,-6.39469921942834));
#11936=CARTESIAN_POINT('Ctrl Pts',(-3.78989358567387,206.607105531561,-6.47480755900256));
#11937=CARTESIAN_POINT('Ctrl Pts',(-3.65809843300235,206.542081286575,-6.55195110329805));
#11938=CARTESIAN_POINT('Ctrl Pts',(-3.52387957064261,206.476959054234,-6.62510554744148));
#11939=CARTESIAN_POINT('Ctrl Pts',(-3.38761165659103,206.411920847683,-6.69406554949809));
#11940=CARTESIAN_POINT('Ctrl Pts',(-3.25136744669109,206.346893954693,-6.76301355578624));
#11941=CARTESIAN_POINT('Ctrl Pts',(-3.11307538411878,206.281951283189,-6.82776836820748));
#11942=CARTESIAN_POINT('Ctrl Pts',(-2.97313145734166,206.217273190525,-6.88817215625554));
#11943=CARTESIAN_POINT('Ctrl Pts',(-2.8331499774231,206.152577741871,-6.94859215330993));
#11944=CARTESIAN_POINT('Ctrl Pts',(-2.69151625970553,206.088147231022,-7.00465866845592));
#11945=CARTESIAN_POINT('Ctrl Pts',(-2.54864063859631,206.02415727582,-7.05626368640968));
#11946=CARTESIAN_POINT('Ctrl Pts',(-2.53215775104539,206.016775056041,-7.06221711430306));
#11947=CARTESIAN_POINT('Ctrl Pts',(-2.51565834512647,206.009398692253,-7.06811121908845));
#11948=CARTESIAN_POINT('Ctrl Pts',(-2.49914305799788,206.002028447915,-7.07394587853976));
#11949=CARTESIAN_POINT('Ctrl Pts',(-2.35598079299498,205.938139708658,-7.12452344682942));
#11950=CARTESIAN_POINT('Ctrl Pts',(-2.21093899485714,205.87379055128,-7.1708721361652));
#11951=CARTESIAN_POINT('Ctrl Pts',(-2.06440202410006,205.809155844927,-7.21281294639894));
#11952=CARTESIAN_POINT('Ctrl Pts',(-1.91225383662799,205.74204613624,-7.25635976072986));
#11953=CARTESIAN_POINT('Ctrl Pts',(-1.75849416561927,205.674628800623,-7.29515405471511));
#11954=CARTESIAN_POINT('Ctrl Pts',(-1.60357741968129,205.607105531561,-7.32904944559231));
#11955=CARTESIAN_POINT('Ctrl Pts',(-1.45439411472333,205.542081286575,-7.36169037413289));
#11956=CARTESIAN_POINT('Ctrl Pts',(-1.30413842461202,205.476959054234,-7.38978847549662));
#11957=CARTESIAN_POINT('Ctrl Pts',(-1.15323012442371,205.411920847683,-7.41326423358633));
#11958=CARTESIAN_POINT('Ctrl Pts',(-1.00234807511963,205.346893954693,-7.43673590800795));
#11959=CARTESIAN_POINT('Ctrl Pts',(-0.850814170352673,205.281951283189,
-7.45558679680064));
#11960=CARTESIAN_POINT('Ctrl Pts',(-0.699053789843954,205.217273190525,
-7.46978916139896));
#11961=CARTESIAN_POINT('Ctrl Pts',(-0.547252685316885,205.152577741871,
-7.48399533711949));
#11962=CARTESIAN_POINT('Ctrl Pts',(-0.39522550915898,205.088147231022,-7.49355053594382));
#11963=CARTESIAN_POINT('Ctrl Pts',(-0.243395891140606,205.02415727582,-7.49847882953766));
#11964=CARTESIAN_POINT('Ctrl Pts',(-0.225880023133996,205.016775056041,
-7.49904738356035));
#11965=CARTESIAN_POINT('Ctrl Pts',(-0.208366777074381,205.009398692253,
-7.49955441349818));
#11966=CARTESIAN_POINT('Ctrl Pts',(-0.190856796705286,205.002028447915,
-7.5));
#11967=CARTESIAN_POINT('Ctrl Pts',(-0.0390720635510205,204.938139708658,
-7.50386255306115));
#11968=CARTESIAN_POINT('Ctrl Pts',(0.113193416374905,204.87379055128,-7.50312239555638));
#11969=CARTESIAN_POINT('Ctrl Pts',(0.265518780411678,204.809155844927,-7.49772806215972));
#11970=CARTESIAN_POINT('Ctrl Pts',(0.42367701122863,204.74204613624,-7.49212716810082));
#11971=CARTESIAN_POINT('Ctrl Pts',(0.581899244411101,204.674628800623,-7.48150838279936));
#11972=CARTESIAN_POINT('Ctrl Pts',(0.739708076930687,204.607105531561,-7.46587290795739));
#11973=CARTESIAN_POINT('Ctrl Pts',(0.891676432865158,204.542081286575,-7.45081609923475));
#11974=CARTESIAN_POINT('Ctrl Pts',(1.04326087688753,204.476959054234,-7.43110741988623));
#11975=CARTESIAN_POINT('Ctrl Pts',(1.19403760735073,204.411920847682,-7.40680096324187));
#11976=CARTESIAN_POINT('Ctrl Pts',(1.34478810981601,204.346893954693,-7.38249873476782));
#11977=CARTESIAN_POINT('Ctrl Pts',(1.49473066238024,204.281951283188,-7.35360044359504));
#11978=CARTESIAN_POINT('Ctrl Pts',(1.64345213319964,204.217273190525,-7.32021115834305));
#11979=CARTESIAN_POINT('Ctrl Pts',(1.79221351256366,204.15257774187,-7.28681291326991));
#11980=CARTESIAN_POINT('Ctrl Pts',(1.93975266792397,204.088147231022,-7.24892146633662));
#11981=CARTESIAN_POINT('Ctrl Pts',(2.08567414198074,204.024157275819,-7.20669061985607));
#11982=CARTESIAN_POINT('Ctrl Pts',(2.1025084152417,204.016775056041,-7.20181864597909));
#11983=CARTESIAN_POINT('Ctrl Pts',(2.1193211828951,204.009398692253,-7.19688896944649));
#11984=CARTESIAN_POINT('Ctrl Pts',(2.13611185762632,204.002028447915,-7.19190186588755));
#11985=CARTESIAN_POINT('Ctrl Pts',(2.28166131170441,203.938139708658,-7.14867131011454));
#11986=CARTESIAN_POINT('Ctrl Pts',(2.42624566734732,203.87379055128,-7.10091475754277));
#11987=CARTESIAN_POINT('Ctrl Pts',(2.56944875671865,203.809155844927,-7.04871331545308));
#11988=CARTESIAN_POINT('Ctrl Pts',(2.71813540129493,203.74204613624,-6.99451296753857));
#11989=CARTESIAN_POINT('Ctrl Pts',(2.86533230206809,203.674628800623,-6.93552054364115));
#11990=CARTESIAN_POINT('Ctrl Pts',(3.01058579312348,203.607105531561,-6.87188471229631));
#11991=CARTESIAN_POINT('Ctrl Pts',(3.15046347852877,203.542081286575,-6.81060403165528));
#11992=CARTESIAN_POINT('Ctrl Pts',(3.28853853492937,203.476959054234,-6.74501779444775));
#11993=CARTESIAN_POINT('Ctrl Pts',(3.42442461876546,203.411920847683,-6.67530840839894));
#11994=CARTESIAN_POINT('Ctrl Pts',(3.56028706487072,203.346893954693,-6.60561114847562));
#11995=CARTESIAN_POINT('Ctrl Pts',(3.69396084347661,203.281951283188,-6.53179244342338));
#11996=CARTESIAN_POINT('Ctrl Pts',(3.82508551084001,203.217273190525,-6.45407988419809));
#11997=CARTESIAN_POINT('Ctrl Pts',(3.95624536474729,203.15257774187,-6.37634647125832));
#11998=CARTESIAN_POINT('Ctrl Pts',(4.08485433881753,203.088147231021,-6.29471745739851));
#11999=CARTESIAN_POINT('Ctrl Pts',(4.21058385833727,203.024157275819,-6.20946132033675));
#12000=CARTESIAN_POINT('Ctrl Pts',(4.22508868089501,203.016775056041,-6.19962572130827));
#12001=CARTESIAN_POINT('Ctrl Pts',(4.23955521930334,203.009398692253,-6.18974188939137));
#12002=CARTESIAN_POINT('Ctrl Pts',(4.25398300016701,203.002028447915,-6.17981026821526));
#12003=CARTESIAN_POINT('Ctrl Pts',(4.37904978050104,202.938139708658,-6.09371831161216));
#12004=CARTESIAN_POINT('Ctrl Pts',(4.50180008775212,202.87379055128,-6.00362010807857));
#12005=CARTESIAN_POINT('Ctrl Pts',(4.62186318631574,202.809155844927,-5.90972139815643));
#12006=CARTESIAN_POINT('Ctrl Pts',(4.74652375991944,202.74204613624,-5.81222710407621));
#12007=CARTESIAN_POINT('Ctrl Pts',(4.86828667005455,202.674628800622,-5.71063563105829));
#12008=CARTESIAN_POINT('Ctrl Pts',(4.98676639590066,202.607105531561,-5.60522856175951));
#12009=CARTESIAN_POINT('Ctrl Pts',(5.10086120834481,202.542081286575,-5.50372258918869));
#12010=CARTESIAN_POINT('Ctrl Pts',(5.21191112857829,202.476959054234,-5.39867883198603));
#12011=CARTESIAN_POINT('Ctrl Pts',(5.319605089128,202.411920847683,-5.29039015693286));
#12012=CARTESIAN_POINT('Ctrl Pts',(5.42728031603811,202.346893954693,-5.1821203189714));
#12013=CARTESIAN_POINT('Ctrl Pts',(5.53160039987475,202.281951283188,-5.07060708921589));
#12014=CARTESIAN_POINT('Ctrl Pts',(5.6322928677404,202.217273190525,-4.95617830277011));
#12015=CARTESIAN_POINT('Ctrl Pts',(5.73301235584613,202.152577741871,-4.84171881002279));
#12016=CARTESIAN_POINT('Ctrl Pts',(5.83010200617296,202.088147231022,-4.72434264585582));
#12017=CARTESIAN_POINT('Ctrl Pts',(5.92333228977606,202.024157275819,-4.60440668292288));
#12018=CARTESIAN_POINT('Ctrl Pts',(5.93408782853791,202.016775056041,-4.59057023570412));
#12019=CARTESIAN_POINT('Ctrl Pts',(5.94479205212776,202.009398692253,-4.57669974673532));
#12020=CARTESIAN_POINT('Ctrl Pts',(5.95544464740895,202.002028447915,-4.56279578422009));
#12021=CARTESIAN_POINT('Ctrl Pts',(6.04778634614835,201.938139708658,-4.44226970733712));
#12022=CARTESIAN_POINT('Ctrl Pts',(6.13668694968221,201.87379055128,-4.31864929275467));
#12023=CARTESIAN_POINT('Ctrl Pts',(6.22185744482191,201.809155844927,-4.19224477495801));
#12024=CARTESIAN_POINT('Ctrl Pts',(6.31028930194743,201.74204613624,-4.06099995549936));
#12025=CARTESIAN_POINT('Ctrl Pts',(6.39469921942835,201.674628800622,-3.92675391456936));
#12026=CARTESIAN_POINT('Ctrl Pts',(6.47480755900257,201.607105531561,-3.78989358567385));
#12027=CARTESIAN_POINT('Ctrl Pts',(6.55195110329815,201.542081286575,-3.65809843300218));
#12028=CARTESIAN_POINT('Ctrl Pts',(6.62510554744167,201.476959054234,-3.52387957064226));
#12029=CARTESIAN_POINT('Ctrl Pts',(6.69406554949835,201.411920847682,-3.38761165659051));
#12030=CARTESIAN_POINT('Ctrl Pts',(6.76301355578675,201.346893954693,-3.25136744669006));
#12031=CARTESIAN_POINT('Ctrl Pts',(6.8277683682082,201.281951283188,-3.11307538411724));
#12032=CARTESIAN_POINT('Ctrl Pts',(6.88817215625643,201.217273190524,-2.97313145733959));
#12033=CARTESIAN_POINT('Ctrl Pts',(6.94859215331078,201.15257774187,-2.83314997742101));
#12034=CARTESIAN_POINT('Ctrl Pts',(7.00465866845674,201.088147231021,-2.69151625970341));
#12035=CARTESIAN_POINT('Ctrl Pts',(7.05626368641046,201.024157275819,-2.54864063859417));
#12036=CARTESIAN_POINT('Ctrl Pts',(7.06221711430357,201.016775056041,-2.53215775104397));
#12037=CARTESIAN_POINT('Ctrl Pts',(7.0681112190887,201.009398692253,-2.51565834512576));
#12038=CARTESIAN_POINT('Ctrl Pts',(7.07394587853975,201.002028447915,-2.49914305799789));
#12039=CARTESIAN_POINT('Ctrl Pts',(7.12452344682944,200.938139708658,-2.35598079299493));
#12040=CARTESIAN_POINT('Ctrl Pts',(7.17087213616524,200.87379055128,-2.21093899485702));
#12041=CARTESIAN_POINT('Ctrl Pts',(7.21281294639899,200.809155844927,-2.06440202409988));
#12042=CARTESIAN_POINT('Ctrl Pts',(7.25635976072991,200.74204613624,-1.91225383662782));
#12043=CARTESIAN_POINT('Ctrl Pts',(7.29515405471514,200.674628800622,-1.75849416561912));
#12044=CARTESIAN_POINT('Ctrl Pts',(7.32904944559233,200.607105531561,-1.60357741968116));
#12045=CARTESIAN_POINT('Ctrl Pts',(7.36169037413292,200.542081286575,-1.45439411472321));
#12046=CARTESIAN_POINT('Ctrl Pts',(7.38978847549664,200.476959054234,-1.30413842461191));
#12047=CARTESIAN_POINT('Ctrl Pts',(7.41326423358634,200.411920847683,-1.15323012442361));
#12048=CARTESIAN_POINT('Ctrl Pts',(7.43673590800806,200.346893954693,-1.00234807511895));
#12049=CARTESIAN_POINT('Ctrl Pts',(7.4555867968008,200.281951283188,-0.850814170351404));
#12050=CARTESIAN_POINT('Ctrl Pts',(7.46978916139914,200.217273190525,-0.699053789842093));
#12051=CARTESIAN_POINT('Ctrl Pts',(7.48399533711963,200.15257774187,-0.547252685315009));
#12052=CARTESIAN_POINT('Ctrl Pts',(7.49355053594392,200.088147231021,-0.395225509157083));
#12053=CARTESIAN_POINT('Ctrl Pts',(7.49847882953772,200.024157275819,-0.243395891138698));
#12054=CARTESIAN_POINT('Ctrl Pts',(7.49904738356038,200.016775056041,-0.225880023132722));
#12055=CARTESIAN_POINT('Ctrl Pts',(7.4995544134982,200.009398692253,-0.208366777073748));
#12056=CARTESIAN_POINT('Ctrl Pts',(7.5,200.002028447915,-0.190856796705287));
#12057=CARTESIAN_POINT('Ctrl Pts',(7.50386255306115,199.938139708658,-0.0390720635509912));
#12058=CARTESIAN_POINT('Ctrl Pts',(7.50312239555638,199.87379055128,0.113193416374972));
#12059=CARTESIAN_POINT('Ctrl Pts',(7.49772806215971,199.809155844927,0.265518780411775));
#12060=CARTESIAN_POINT('Ctrl Pts',(7.49212716810081,199.74204613624,0.423677011228717));
#12061=CARTESIAN_POINT('Ctrl Pts',(7.48150838279936,199.674628800623,0.581899244411163));
#12062=CARTESIAN_POINT('Ctrl Pts',(7.46587290795738,199.607105531561,0.73970807693074));
#12063=CARTESIAN_POINT('Ctrl Pts',(7.4508160992348,199.542081286575,0.891676432864664));
#12064=CARTESIAN_POINT('Ctrl Pts',(7.43110741988637,199.476959054234,1.04326087688649));
#12065=CARTESIAN_POINT('Ctrl Pts',(7.40680096324213,199.411920847683,1.19403760734915));
#12066=CARTESIAN_POINT('Ctrl Pts',(7.38249873476819,199.346893954694,1.34478810981391));
#12067=CARTESIAN_POINT('Ctrl Pts',(7.35360044359557,199.281951283189,1.49473066237762));
#12068=CARTESIAN_POINT('Ctrl Pts',(7.32021115834376,199.217273190526,1.64345213319651));
#12069=CARTESIAN_POINT('Ctrl Pts',(7.28681291327069,199.152577741872,1.79221351256049));
#12070=CARTESIAN_POINT('Ctrl Pts',(7.24892146633748,199.088147231023,1.93975266792075));
#12071=CARTESIAN_POINT('Ctrl Pts',(7.20669061985702,199.02415727582,2.08567414197748));
#12072=CARTESIAN_POINT('Ctrl Pts',(7.20181864597973,199.016775056042,2.10250841523952));
#12073=CARTESIAN_POINT('Ctrl Pts',(7.19688896944681,199.009398692254,2.11932118289401));
#12074=CARTESIAN_POINT('Ctrl Pts',(7.19190186588755,199.002028447915,2.13611185762632));
#12075=CARTESIAN_POINT('Ctrl Pts',(7.14867131011454,198.938139708658,2.28166131170442));
#12076=CARTESIAN_POINT('Ctrl Pts',(7.10091475754276,198.87379055128,2.42624566734735));
#12077=CARTESIAN_POINT('Ctrl Pts',(7.04871331545307,198.809155844927,2.56944875671869));
#12078=CARTESIAN_POINT('Ctrl Pts',(6.99451296753856,198.74204613624,2.71813540129497));
#12079=CARTESIAN_POINT('Ctrl Pts',(6.93552054364114,198.674628800622,2.86533230206812));
#12080=CARTESIAN_POINT('Ctrl Pts',(6.8718847122963,198.607105531561,3.0105857931235));
#12081=CARTESIAN_POINT('Ctrl Pts',(6.81060403165536,198.542081286575,3.1504634785286));
#12082=CARTESIAN_POINT('Ctrl Pts',(6.74501779444792,198.476959054234,3.288538534929));
#12083=CARTESIAN_POINT('Ctrl Pts',(6.67530840839923,198.411920847683,3.42442461876491));
#12084=CARTESIAN_POINT('Ctrl Pts',(6.60561114847646,198.346893954694,3.56028706486911));
#12085=CARTESIAN_POINT('Ctrl Pts',(6.53179244342483,198.281951283189,3.69396084347398));
#12086=CARTESIAN_POINT('Ctrl Pts',(6.45407988420023,198.217273190526,3.8250855108364));
#12087=CARTESIAN_POINT('Ctrl Pts',(6.37634647126055,198.152577741872,3.9562453647437));
#12088=CARTESIAN_POINT('Ctrl Pts',(6.29471745740083,198.088147231023,4.08485433881396));
#12089=CARTESIAN_POINT('Ctrl Pts',(6.20946132033916,198.024157275821,4.21058385833372));
#12090=CARTESIAN_POINT('Ctrl Pts',(6.19962572130989,198.016775056042,4.22508868089265));
#12091=CARTESIAN_POINT('Ctrl Pts',(6.18974188939218,198.009398692254,4.23955521930217));
#12092=CARTESIAN_POINT('Ctrl Pts',(6.17981026821526,198.002028447915,4.25398300016701));
#12093=CARTESIAN_POINT('Ctrl Pts',(6.09371831161217,197.938139708658,4.37904978050101));
#12094=CARTESIAN_POINT('Ctrl Pts',(6.0036201080786,197.87379055128,4.50180008775207));
#12095=CARTESIAN_POINT('Ctrl Pts',(5.90972139815648,197.809155844927,4.62186318631566));
#12096=CARTESIAN_POINT('Ctrl Pts',(5.81222710407627,197.74204613624,4.74652375991938));
#12097=CARTESIAN_POINT('Ctrl Pts',(5.71063563105834,197.674628800623,4.86828667005449));
#12098=CARTESIAN_POINT('Ctrl Pts',(5.60522856175956,197.607105531561,4.9867663959006));
#12099=CARTESIAN_POINT('Ctrl Pts',(5.50372258918911,197.542081286575,5.10086120834435));
#12100=CARTESIAN_POINT('Ctrl Pts',(5.39867883198685,197.476959054235,5.21191112857743));
#12101=CARTESIAN_POINT('Ctrl Pts',(5.29039015693409,197.411920847683,5.31960508912677));
#12102=CARTESIAN_POINT('Ctrl Pts',(5.18212031897387,197.346893954695,5.4272803160357));
#12103=CARTESIAN_POINT('Ctrl Pts',(5.07060708921967,197.281951283191,5.53160039987124));
#12104=CARTESIAN_POINT('Ctrl Pts',(4.95617830277527,197.217273190528,5.63229286773586));
#12105=CARTESIAN_POINT('Ctrl Pts',(4.84171881002731,197.152577741873,5.73301235584234));
#12106=CARTESIAN_POINT('Ctrl Pts',(4.72434264585968,197.088147231024,5.83010200616986));
#12107=CARTESIAN_POINT('Ctrl Pts',(4.60440668292603,197.024157275821,5.92333228977361));
#12108=CARTESIAN_POINT('Ctrl Pts',(4.59057023570623,197.016775056042,5.93408782853628));
#12109=CARTESIAN_POINT('Ctrl Pts',(4.57669974673637,197.009398692254,5.94479205212695));
#12110=CARTESIAN_POINT('Ctrl Pts',(4.56279578422009,197.002028447915,5.95544464740895));
#12111=CARTESIAN_POINT('Ctrl Pts',(4.44226970733712,196.938139708658,6.04778634614835));
#12112=CARTESIAN_POINT('Ctrl Pts',(4.31864929275467,196.87379055128,6.13668694968221));
#12113=CARTESIAN_POINT('Ctrl Pts',(4.19224477495802,196.809155844927,6.22185744482191));
#12114=CARTESIAN_POINT('Ctrl Pts',(4.06099995549936,196.74204613624,6.31028930194743));
#12115=CARTESIAN_POINT('Ctrl Pts',(3.92675391456935,196.674628800622,6.39469921942835));
#12116=CARTESIAN_POINT('Ctrl Pts',(3.78989358567384,196.607105531561,6.47480755900257));
#12117=CARTESIAN_POINT('Ctrl Pts',(3.6580984330025,196.542081286575,6.55195110329796));
#12118=CARTESIAN_POINT('Ctrl Pts',(3.52387957064293,196.476959054234,6.62510554744131));
#12119=CARTESIAN_POINT('Ctrl Pts',(3.38761165659153,196.411920847683,6.69406554949784));
#12120=CARTESIAN_POINT('Ctrl Pts',(3.25136744669109,196.346893954693,6.76301355578625));
#12121=CARTESIAN_POINT('Ctrl Pts',(3.11307538411827,196.281951283188,6.82776836820773));
#12122=CARTESIAN_POINT('Ctrl Pts',(2.97313145734063,196.217273190525,6.88817215625598));
#12123=CARTESIAN_POINT('Ctrl Pts',(2.83314997742163,196.15257774187,6.94859215331054));
#12124=CARTESIAN_POINT('Ctrl Pts',(2.69151625970362,196.088147231021,7.00465866845667));
#12125=CARTESIAN_POINT('Ctrl Pts',(2.54864063859395,196.024157275819,7.05626368641054));
#12126=CARTESIAN_POINT('Ctrl Pts',(2.53215775104383,196.016775056041,7.06221711430362));
#12127=CARTESIAN_POINT('Ctrl Pts',(2.51565834512569,196.009398692253,7.06811121908872));
#12128=CARTESIAN_POINT('Ctrl Pts',(2.49914305799789,196.002028447915,7.07394587853975));
#12129=CARTESIAN_POINT('Ctrl Pts',(2.35598079299495,195.938139708658,7.12452344682943));
#12130=CARTESIAN_POINT('Ctrl Pts',(2.21093899485708,195.87379055128,7.17087213616522));
#12131=CARTESIAN_POINT('Ctrl Pts',(2.06440202409996,195.809155844927,7.21281294639897));
#12132=CARTESIAN_POINT('Ctrl Pts',(1.9122538366279,195.74204613624,7.25635976072989));
#12133=CARTESIAN_POINT('Ctrl Pts',(1.75849416561919,195.674628800623,7.29515405471513));
#12134=CARTESIAN_POINT('Ctrl Pts',(1.60357741968122,195.607105531561,7.32904944559232));
#12135=CARTESIAN_POINT('Ctrl Pts',(1.4543941147231,195.542081286575,7.36169037413294));
#12136=CARTESIAN_POINT('Ctrl Pts',(1.30413842461163,195.476959054234,7.38978847549669));
#12137=CARTESIAN_POINT('Ctrl Pts',(1.15323012442317,195.411920847683,7.41326423358641));
#12138=CARTESIAN_POINT('Ctrl Pts',(1.00234807511844,195.346893954693,7.43673590800813));
#12139=CARTESIAN_POINT('Ctrl Pts',(0.850814170350841,195.281951283188,7.45558679680086));
#12140=CARTESIAN_POINT('Ctrl Pts',(0.69905378984147,195.217273190524,7.46978916139919));
#12141=CARTESIAN_POINT('Ctrl Pts',(0.547252685314392,195.15257774187,7.48399533711967));
#12142=CARTESIAN_POINT('Ctrl Pts',(0.395225509156497,195.088147231021,7.49355053594395));
#12143=CARTESIAN_POINT('Ctrl Pts',(0.243395891138119,195.024157275819,7.49847882953774));
#12144=CARTESIAN_POINT('Ctrl Pts',(0.225880023132343,195.016775056041,7.4990473835604));
#12145=CARTESIAN_POINT('Ctrl Pts',(0.208366777073546,195.009398692253,7.49955441349821));
#12146=CARTESIAN_POINT('Ctrl Pts',(0.190856796705285,195.002028447915,7.5));
#12147=CARTESIAN_POINT('Ctrl Pts',(0.127311648028404,194.975281229334,7.50161706980302));
#12148=CARTESIAN_POINT('Ctrl Pts',(0.0636823578853578,194.948453397593,
7.50242803155527));
#12149=CARTESIAN_POINT('Ctrl Pts',(-4.06843965232862E-7,194.921557632927,
7.50242802810186));
#12150=CARTESIAN_POINT('Origin',(0.,240.,0.));
#12151=CARTESIAN_POINT('Ctrl Pts',(5.38002895896315E-16,217.99585953923,
7.50000000439337));
#12152=CARTESIAN_POINT('Ctrl Pts',(-1.18775172812189,217.495912211348,7.50000000439337));
#12153=CARTESIAN_POINT('Ctrl Pts',(-2.317383311169,216.995967593475,7.13300320026677));
#12154=CARTESIAN_POINT('Ctrl Pts',(-3.44714003087638,216.495967593475,6.76596574150984));
#12155=CARTESIAN_POINT('Ctrl Pts',(-4.40818170865423,215.995967593475,6.06777834873578));
#12156=CARTESIAN_POINT('Ctrl Pts',(-5.36922338643209,215.495967593475,5.36959095596173));
#12157=CARTESIAN_POINT('Ctrl Pts',(-6.06747656688843,214.995967593475,4.40859707573286));
#12158=CARTESIAN_POINT('Ctrl Pts',(-6.76572974734476,214.495967593475,3.447603195504));
#12159=CARTESIAN_POINT('Ctrl Pts',(-7.13284454416054,213.995967593475,2.31787160445521));
#12160=CARTESIAN_POINT('Ctrl Pts',(-7.49995934097631,213.495967593475,1.18814001340642));
#12161=CARTESIAN_POINT('Ctrl Pts',(-7.5,212.995967593475,0.000256710972401669));
#12162=CARTESIAN_POINT('Ctrl Pts',(-7.50004065902369,212.495967593475,-1.18762659146162));
#12163=CARTESIAN_POINT('Ctrl Pts',(-7.13300320026677,211.995967593475,-2.317383311169));
#12164=CARTESIAN_POINT('Ctrl Pts',(-6.76596574150984,211.495967593475,-3.44714003087638));
#12165=CARTESIAN_POINT('Ctrl Pts',(-6.06777834873578,210.995967593475,-4.40818170865423));
#12166=CARTESIAN_POINT('Ctrl Pts',(-5.36959095596173,210.495967593475,-5.36922338643209));
#12167=CARTESIAN_POINT('Ctrl Pts',(-4.40859707573286,209.995967593475,-6.06747656688843));
#12168=CARTESIAN_POINT('Ctrl Pts',(-3.447603195504,209.495967593475,-6.76572974734476));
#12169=CARTESIAN_POINT('Ctrl Pts',(-2.31787160445521,208.995967593475,-7.13284454416054));
#12170=CARTESIAN_POINT('Ctrl Pts',(-1.18814001340642,208.495967593475,-7.49995934097631));
#12171=CARTESIAN_POINT('Ctrl Pts',(-0.000256710972402128,207.995967593475,
-7.5));
#12172=CARTESIAN_POINT('Ctrl Pts',(1.18762659146162,207.495967593475,-7.50004065902369));
#12173=CARTESIAN_POINT('Ctrl Pts',(2.317383311169,206.995967593475,-7.13300320026677));
#12174=CARTESIAN_POINT('Ctrl Pts',(3.44714003087638,206.495967593475,-6.76596574150984));
#12175=CARTESIAN_POINT('Ctrl Pts',(4.40818170865423,205.995967593475,-6.06777834873578));
#12176=CARTESIAN_POINT('Ctrl Pts',(5.36922338643209,205.495967593475,-5.36959095596173));
#12177=CARTESIAN_POINT('Ctrl Pts',(6.06747656688843,204.995967593475,-4.40859707573286));
#12178=CARTESIAN_POINT('Ctrl Pts',(6.76572974734476,204.495967593475,-3.447603195504));
#12179=CARTESIAN_POINT('Ctrl Pts',(7.13284454416054,203.995967593475,-2.31787160445521));
#12180=CARTESIAN_POINT('Ctrl Pts',(7.49995934097631,203.495967593475,-1.18814001340642));
#12181=CARTESIAN_POINT('Ctrl Pts',(7.5,202.995967593475,-0.000256710972402588));
#12182=CARTESIAN_POINT('Ctrl Pts',(7.50004065902369,202.495967593475,1.18762659146162));
#12183=CARTESIAN_POINT('Ctrl Pts',(7.13300320026677,201.995967593475,2.317383311169));
#12184=CARTESIAN_POINT('Ctrl Pts',(6.76596574150984,201.495967593475,3.44714003087638));
#12185=CARTESIAN_POINT('Ctrl Pts',(6.06777834873579,200.995967593475,4.40818170865423));
#12186=CARTESIAN_POINT('Ctrl Pts',(5.36959095596173,200.495967593475,5.36922338643209));
#12187=CARTESIAN_POINT('Ctrl Pts',(4.40859707573286,199.995967593475,6.06747656688843));
#12188=CARTESIAN_POINT('Ctrl Pts',(3.447603195504,199.495967593475,6.76572974734476));
#12189=CARTESIAN_POINT('Ctrl Pts',(2.31787160445521,198.995967593475,7.13284454416054));
#12190=CARTESIAN_POINT('Ctrl Pts',(1.18814001340643,198.495967593475,7.49995934097631));
#12191=CARTESIAN_POINT('Ctrl Pts',(0.00025671097240121,197.995967593475,
7.5));
#12192=CARTESIAN_POINT('Ctrl Pts',(0.000128355486237033,197.995913566499,
7.50000000439337));
#12193=CARTESIAN_POINT('Ctrl Pts',(5.38866871829646E-16,197.99585953923,
7.50000000439337));
#12194=CARTESIAN_POINT('Ctrl Pts',(-4.06843934450864E-7,234.921557632927,
7.50242802810186));
#12195=CARTESIAN_POINT('Ctrl Pts',(-0.152090385416014,234.857323985265,
7.50242801985428));
#12196=CARTESIAN_POINT('Ctrl Pts',(-0.304485788638578,234.792702491972,
7.49779895914527));
#12197=CARTESIAN_POINT('Ctrl Pts',(-0.456762644215501,234.72787053402,7.48851081348607));
#12198=CARTESIAN_POINT('Ctrl Pts',(-0.609070650331329,234.663025313709,
7.4792207677959));
#12199=CARTESIAN_POINT('Ctrl Pts',(-0.761259533138642,234.597969762788,
7.46526968655066));
#12200=CARTESIAN_POINT('Ctrl Pts',(-0.912902720439174,234.532885263597,
7.44667945730601));
#12201=CARTESIAN_POINT('Ctrl Pts',(-1.06450493068721,234.467818351553,7.42809425151684));
#12202=CARTESIAN_POINT('Ctrl Pts',(-1.2155612127989,234.402722732839,7.40487246128567));
#12203=CARTESIAN_POINT('Ctrl Pts',(-1.36565093134662,234.3377801784,7.3770877621566));
#12204=CARTESIAN_POINT('Ctrl Pts',(-1.51579830432564,234.272812677376,7.34929239000448));
#12205=CARTESIAN_POINT('Ctrl Pts',(-1.66497786162574,234.207998581557,7.31693074896052));
#12206=CARTESIAN_POINT('Ctrl Pts',(-1.81278187771317,234.143517028959,7.28012693437987));
#12207=CARTESIAN_POINT('Ctrl Pts',(-1.92135204017761,234.096151789321,7.25309251248725));
#12208=CARTESIAN_POINT('Ctrl Pts',(-2.02918025203209,234.04896593395,7.22366229239563));
#12209=CARTESIAN_POINT('Ctrl Pts',(-2.13611185762633,234.002028447915,7.19190186588755));
#12210=CARTESIAN_POINT('Ctrl Pts',(-2.28166131170441,233.938139708658,7.14867131011454));
#12211=CARTESIAN_POINT('Ctrl Pts',(-2.42624566734732,233.87379055128,7.10091475754277));
#12212=CARTESIAN_POINT('Ctrl Pts',(-2.56944875671866,233.809155844927,7.04871331545308));
#12213=CARTESIAN_POINT('Ctrl Pts',(-2.71813540129493,233.74204613624,6.99451296753857));
#12214=CARTESIAN_POINT('Ctrl Pts',(-2.8653323020681,233.674628800622,6.93552054364115));
#12215=CARTESIAN_POINT('Ctrl Pts',(-3.01058579312348,233.607105531561,6.8718847122963));
#12216=CARTESIAN_POINT('Ctrl Pts',(-3.15046347852879,233.542081286575,6.81060403165527));
#12217=CARTESIAN_POINT('Ctrl Pts',(-3.28853853492939,233.476959054234,6.74501779444774));
#12218=CARTESIAN_POINT('Ctrl Pts',(-3.42442461876549,233.411920847683,6.67530840839893));
#12219=CARTESIAN_POINT('Ctrl Pts',(-3.56028706487034,233.346893954693,6.60561114847581));
#12220=CARTESIAN_POINT('Ctrl Pts',(-3.69396084347583,233.281951283188,6.5317924434238));
#12221=CARTESIAN_POINT('Ctrl Pts',(-3.82508551083885,233.217273190525,6.45407988419878));
#12222=CARTESIAN_POINT('Ctrl Pts',(-3.95624536474616,233.152577741871,6.37634647125902));
#12223=CARTESIAN_POINT('Ctrl Pts',(-4.08485433881642,233.088147231022,6.29471745739923));
#12224=CARTESIAN_POINT('Ctrl Pts',(-4.21058385833618,233.024157275819,6.20946132033749));
#12225=CARTESIAN_POINT('Ctrl Pts',(-4.22508868089429,233.016775056041,6.19962572130877));
#12226=CARTESIAN_POINT('Ctrl Pts',(-4.23955521930298,233.009398692253,6.18974188939162));
#12227=CARTESIAN_POINT('Ctrl Pts',(-4.25398300016701,233.002028447915,6.17981026821526));
#12228=CARTESIAN_POINT('Ctrl Pts',(-4.3790497805011,232.938139708658,6.09371831161211));
#12229=CARTESIAN_POINT('Ctrl Pts',(-4.50180008775226,232.87379055128,6.00362010807847));
#12230=CARTESIAN_POINT('Ctrl Pts',(-4.62186318631593,232.809155844927,5.90972139815627));
#12231=CARTESIAN_POINT('Ctrl Pts',(-4.74652375991963,232.74204613624,5.81222710407607));
#12232=CARTESIAN_POINT('Ctrl Pts',(-4.86828667005471,232.674628800622,5.71063563105815));
#12233=CARTESIAN_POINT('Ctrl Pts',(-4.9867663959008,232.607105531561,5.60522856175938));
#12234=CARTESIAN_POINT('Ctrl Pts',(-5.10086120834483,232.542081286575,5.50372258918868));
#12235=CARTESIAN_POINT('Ctrl Pts',(-5.21191112857818,232.476959054234,5.39867883198613));
#12236=CARTESIAN_POINT('Ctrl Pts',(-5.31960508912778,232.411920847683,5.29039015693308));
#12237=CARTESIAN_POINT('Ctrl Pts',(-5.4272803160379,232.346893954693,5.18212031897162));
#12238=CARTESIAN_POINT('Ctrl Pts',(-5.53160039987455,232.281951283189,5.07060708921611));
#12239=CARTESIAN_POINT('Ctrl Pts',(-5.63229286774021,232.217273190525,4.95617830277033));
#12240=CARTESIAN_POINT('Ctrl Pts',(-5.7330123558459,232.152577741871,4.84171881002306));
#12241=CARTESIAN_POINT('Ctrl Pts',(-5.83010200617269,232.088147231022,4.72434264585615));
#12242=CARTESIAN_POINT('Ctrl Pts',(-5.92333228977576,232.02415727582,4.60440668292327));
#12243=CARTESIAN_POINT('Ctrl Pts',(-5.9340878285377,232.016775056041,4.59057023570438));
#12244=CARTESIAN_POINT('Ctrl Pts',(-5.94479205212766,232.009398692253,4.57669974673544));
#12245=CARTESIAN_POINT('Ctrl Pts',(-5.95544464740896,232.002028447915,4.56279578422008));
#12246=CARTESIAN_POINT('Ctrl Pts',(-6.04778634614836,231.938139708658,4.44226970733711));
#12247=CARTESIAN_POINT('Ctrl Pts',(-6.13668694968222,231.87379055128,4.31864929275465));
#12248=CARTESIAN_POINT('Ctrl Pts',(-6.22185744482192,231.809155844927,4.192244774958));
#12249=CARTESIAN_POINT('Ctrl Pts',(-6.31028930194744,231.74204613624,4.06099995549935));
#12250=CARTESIAN_POINT('Ctrl Pts',(-6.39469921942836,231.674628800622,3.92675391456934));
#12251=CARTESIAN_POINT('Ctrl Pts',(-6.47480755900258,231.607105531561,3.78989358567383));
#12252=CARTESIAN_POINT('Ctrl Pts',(-6.55195110329806,231.542081286575,3.65809843300233));
#12253=CARTESIAN_POINT('Ctrl Pts',(-6.62510554744149,231.476959054234,3.52387957064259));
#12254=CARTESIAN_POINT('Ctrl Pts',(-6.6940655494981,231.411920847683,3.38761165659102));
#12255=CARTESIAN_POINT('Ctrl Pts',(-6.76301355578627,231.346893954693,3.25136744669103));
#12256=CARTESIAN_POINT('Ctrl Pts',(-6.82776836820753,231.281951283188,3.11307538411867));
#12257=CARTESIAN_POINT('Ctrl Pts',(-6.8881721562556,231.217273190525,2.97313145734151));
#12258=CARTESIAN_POINT('Ctrl Pts',(-6.94859215330999,231.152577741871,2.83314997742295));
#12259=CARTESIAN_POINT('Ctrl Pts',(-7.00465866845598,231.088147231022,2.69151625970537));
#12260=CARTESIAN_POINT('Ctrl Pts',(-7.05626368640974,231.024157275819,2.54864063859615));
#12261=CARTESIAN_POINT('Ctrl Pts',(-7.06221711430309,231.016775056041,2.53215775104529));
#12262=CARTESIAN_POINT('Ctrl Pts',(-7.06811121908846,231.009398692253,2.51565834512643));
#12263=CARTESIAN_POINT('Ctrl Pts',(-7.07394587853975,231.002028447915,2.49914305799789));
#12264=CARTESIAN_POINT('Ctrl Pts',(-7.12452344682943,230.938139708658,2.35598079299495));
#12265=CARTESIAN_POINT('Ctrl Pts',(-7.17087213616522,230.87379055128,2.21093899485707));
#12266=CARTESIAN_POINT('Ctrl Pts',(-7.21281294639897,230.809155844927,2.06440202409995));
#12267=CARTESIAN_POINT('Ctrl Pts',(-7.25635976072989,230.74204613624,1.91225383662789));
#12268=CARTESIAN_POINT('Ctrl Pts',(-7.29515405471513,230.674628800623,1.75849416561917));
#12269=CARTESIAN_POINT('Ctrl Pts',(-7.32904944559233,230.607105531561,1.6035774196812));
#12270=CARTESIAN_POINT('Ctrl Pts',(-7.36169037413292,230.542081286575,1.45439411472321));
#12271=CARTESIAN_POINT('Ctrl Pts',(-7.38978847549665,230.476959054234,1.30413842461186));
#12272=CARTESIAN_POINT('Ctrl Pts',(-7.41326423358636,230.411920847683,1.15323012442351));
#12273=CARTESIAN_POINT('Ctrl Pts',(-7.43673590800799,230.346893954693,1.00234807511941));
#12274=CARTESIAN_POINT('Ctrl Pts',(-7.45558679680067,230.281951283188,0.850814170352427));
#12275=CARTESIAN_POINT('Ctrl Pts',(-7.46978916139899,230.217273190525,0.699053789843682));
#12276=CARTESIAN_POINT('Ctrl Pts',(-7.48399533711951,230.152577741871,0.547252685316623));
#12277=CARTESIAN_POINT('Ctrl Pts',(-7.49355053594384,230.088147231022,0.395225509158728));
#12278=CARTESIAN_POINT('Ctrl Pts',(-7.49847882953767,230.02415727582,0.243395891140365));
#12279=CARTESIAN_POINT('Ctrl Pts',(-7.49904738356035,230.016775056041,0.225880023133833));
#12280=CARTESIAN_POINT('Ctrl Pts',(-7.49955441349819,230.009398692253,0.208366777074296));
#12281=CARTESIAN_POINT('Ctrl Pts',(-7.5,230.002028447915,0.19085679670528));
#12282=CARTESIAN_POINT('Ctrl Pts',(-7.50386255306115,229.938139708658,0.0390720635509798));
#12283=CARTESIAN_POINT('Ctrl Pts',(-7.50312239555638,229.87379055128,-0.113193416374988));
#12284=CARTESIAN_POINT('Ctrl Pts',(-7.49772806215971,229.809155844927,-0.265518780411795));
#12285=CARTESIAN_POINT('Ctrl Pts',(-7.49212716810081,229.74204613624,-0.423677011228737));
#12286=CARTESIAN_POINT('Ctrl Pts',(-7.48150838279935,229.674628800622,-0.581899244411182));
#12287=CARTESIAN_POINT('Ctrl Pts',(-7.46587290795738,229.607105531561,-0.739708076930759));
#12288=CARTESIAN_POINT('Ctrl Pts',(-7.4508160992348,229.542081286575,-0.891676432864674));
#12289=CARTESIAN_POINT('Ctrl Pts',(-7.43110741988637,229.476959054234,-1.0432608768865));
#12290=CARTESIAN_POINT('Ctrl Pts',(-7.40680096324213,229.411920847683,-1.19403760734915));
#12291=CARTESIAN_POINT('Ctrl Pts',(-7.38249873476809,229.346893954693,-1.34478810981454));
#12292=CARTESIAN_POINT('Ctrl Pts',(-7.35360044359533,229.281951283189,-1.49473066237887));
#12293=CARTESIAN_POINT('Ctrl Pts',(-7.32021115834334,229.217273190525,-1.64345213319836));
#12294=CARTESIAN_POINT('Ctrl Pts',(-7.28681291327022,229.152577741871,-1.79221351256241));
#12295=CARTESIAN_POINT('Ctrl Pts',(-7.24892146633694,229.088147231022,-1.93975266792275));
#12296=CARTESIAN_POINT('Ctrl Pts',(-7.20669061985642,229.02415727582,-2.08567414197955));
#12297=CARTESIAN_POINT('Ctrl Pts',(-7.20181864597933,229.016775056041,-2.1025084152409));
#12298=CARTESIAN_POINT('Ctrl Pts',(-7.19688896944661,229.009398692253,-2.1193211828947));
#12299=CARTESIAN_POINT('Ctrl Pts',(-7.19190186588755,229.002028447915,-2.13611185762632));
#12300=CARTESIAN_POINT('Ctrl Pts',(-7.14867131011454,228.938139708658,-2.28166131170441));
#12301=CARTESIAN_POINT('Ctrl Pts',(-7.10091475754277,228.87379055128,-2.42624566734733));
#12302=CARTESIAN_POINT('Ctrl Pts',(-7.04871331545307,228.809155844927,-2.56944875671868));
#12303=CARTESIAN_POINT('Ctrl Pts',(-6.99451296753857,228.74204613624,-2.71813540129495));
#12304=CARTESIAN_POINT('Ctrl Pts',(-6.93552054364114,228.674628800622,-2.86533230206812));
#12305=CARTESIAN_POINT('Ctrl Pts',(-6.8718847122963,228.607105531561,-3.0105857931235));
#12306=CARTESIAN_POINT('Ctrl Pts',(-6.81060403165529,228.542081286575,-3.15046347852874));
#12307=CARTESIAN_POINT('Ctrl Pts',(-6.74501779444778,228.476959054234,-3.2885385349293));
#12308=CARTESIAN_POINT('Ctrl Pts',(-6.675308408399,228.411920847683,-3.42442461876534));
#12309=CARTESIAN_POINT('Ctrl Pts',(-6.60561114847594,228.346893954693,-3.5602870648701));
#12310=CARTESIAN_POINT('Ctrl Pts',(-6.53179244342398,228.281951283189,-3.69396084347551));
#12311=CARTESIAN_POINT('Ctrl Pts',(-6.45407988419902,228.217273190525,-3.82508551083845));
#12312=CARTESIAN_POINT('Ctrl Pts',(-6.37634647125928,228.152577741871,-3.95624536474574));
#12313=CARTESIAN_POINT('Ctrl Pts',(-6.29471745739952,228.088147231022,-4.08485433881598));
#12314=CARTESIAN_POINT('Ctrl Pts',(-6.2094613203378,228.02415727582,-4.21058385833573));
#12315=CARTESIAN_POINT('Ctrl Pts',(-6.19962572130897,228.016775056041,-4.22508868089399));
#12316=CARTESIAN_POINT('Ctrl Pts',(-6.18974188939172,228.009398692253,-4.23955521930283));
#12317=CARTESIAN_POINT('Ctrl Pts',(-6.17981026821526,228.002028447915,-4.25398300016701));
#12318=CARTESIAN_POINT('Ctrl Pts',(-6.09371831161215,227.938139708658,-4.37904978050104));
#12319=CARTESIAN_POINT('Ctrl Pts',(-6.00362010807856,227.87379055128,-4.50180008775213));
#12320=CARTESIAN_POINT('Ctrl Pts',(-5.90972139815641,227.809155844927,-4.62186318631575));
#12321=CARTESIAN_POINT('Ctrl Pts',(-5.8122271040762,227.74204613624,-4.74652375991946));
#12322=CARTESIAN_POINT('Ctrl Pts',(-5.71063563105828,227.674628800622,-4.86828667005456));
#12323=CARTESIAN_POINT('Ctrl Pts',(-5.6052285617595,227.607105531561,-4.98676639590066));
#12324=CARTESIAN_POINT('Ctrl Pts',(-5.50372258918886,227.542081286575,-5.10086120834462));
#12325=CARTESIAN_POINT('Ctrl Pts',(-5.39867883198638,227.476959054234,-5.21191112857791));
#12326=CARTESIAN_POINT('Ctrl Pts',(-5.29039015693341,227.411920847683,-5.31960508912745));
#12327=CARTESIAN_POINT('Ctrl Pts',(-5.18212031897197,227.346893954694,-5.42728031603756));
#12328=CARTESIAN_POINT('Ctrl Pts',(-5.07060708921648,227.281951283189,-5.5316003998742));
#12329=CARTESIAN_POINT('Ctrl Pts',(-4.95617830277073,227.217273190526,-5.63229286773986));
#12330=CARTESIAN_POINT('Ctrl Pts',(-4.84171881002346,227.152577741871,-5.73301235584555));
#12331=CARTESIAN_POINT('Ctrl Pts',(-4.72434264585657,227.088147231022,-5.83010200617235));
#12332=CARTESIAN_POINT('Ctrl Pts',(-4.60440668292369,227.02415727582,-5.92333228977543));
#12333=CARTESIAN_POINT('Ctrl Pts',(-4.59057023570467,227.016775056041,-5.93408782853748));
#12334=CARTESIAN_POINT('Ctrl Pts',(-4.57669974673559,227.009398692253,-5.94479205212755));
#12335=CARTESIAN_POINT('Ctrl Pts',(-4.56279578422009,227.002028447915,-5.95544464740895));
#12336=CARTESIAN_POINT('Ctrl Pts',(-4.44226970733717,226.938139708658,-6.04778634614832));
#12337=CARTESIAN_POINT('Ctrl Pts',(-4.31864929275475,226.87379055128,-6.13668694968215));
#12338=CARTESIAN_POINT('Ctrl Pts',(-4.19224477495815,226.809155844927,-6.22185744482182));
#12339=CARTESIAN_POINT('Ctrl Pts',(-4.06099995549949,226.74204613624,-6.31028930194735));
#12340=CARTESIAN_POINT('Ctrl Pts',(-3.92675391456947,226.674628800623,-6.39469921942828));
#12341=CARTESIAN_POINT('Ctrl Pts',(-3.78989358567395,226.607105531561,-6.47480755900251));
#12342=CARTESIAN_POINT('Ctrl Pts',(-3.65809843300246,226.542081286575,-6.55195110329799));
#12343=CARTESIAN_POINT('Ctrl Pts',(-3.52387957064274,226.476959054234,-6.62510554744141));
#12344=CARTESIAN_POINT('Ctrl Pts',(-3.38761165659118,226.411920847683,-6.69406554949802));
#12345=CARTESIAN_POINT('Ctrl Pts',(-3.25136744669125,226.346893954693,-6.76301355578616));
#12346=CARTESIAN_POINT('Ctrl Pts',(-3.11307538411895,226.281951283189,-6.8277683682074));
#12347=CARTESIAN_POINT('Ctrl Pts',(-2.97313145734185,226.217273190525,-6.88817215625545));
#12348=CARTESIAN_POINT('Ctrl Pts',(-2.83314997742316,226.152577741871,-6.94859215330991));
#12349=CARTESIAN_POINT('Ctrl Pts',(-2.69151625970544,226.088147231022,-7.00465866845596));
#12350=CARTESIAN_POINT('Ctrl Pts',(-2.54864063859608,226.024157275819,-7.05626368640977));
#12351=CARTESIAN_POINT('Ctrl Pts',(-2.53215775104524,226.016775056041,-7.06221711430311));
#12352=CARTESIAN_POINT('Ctrl Pts',(-2.5156583451264,226.009398692253,-7.06811121908847));
#12353=CARTESIAN_POINT('Ctrl Pts',(-2.49914305799788,226.002028447915,-7.07394587853975));
#12354=CARTESIAN_POINT('Ctrl Pts',(-2.35598079299495,225.938139708658,-7.12452344682943));
#12355=CARTESIAN_POINT('Ctrl Pts',(-2.21093899485708,225.87379055128,-7.17087213616522));
#12356=CARTESIAN_POINT('Ctrl Pts',(-2.06440202409996,225.809155844927,-7.21281294639897));
#12357=CARTESIAN_POINT('Ctrl Pts',(-1.9122538366279,225.74204613624,-7.25635976072989));
#12358=CARTESIAN_POINT('Ctrl Pts',(-1.75849416561919,225.674628800623,-7.29515405471513));
#12359=CARTESIAN_POINT('Ctrl Pts',(-1.60357741968122,225.607105531561,-7.32904944559232));
#12360=CARTESIAN_POINT('Ctrl Pts',(-1.45439411472326,225.542081286575,-7.36169037413291));
#12361=CARTESIAN_POINT('Ctrl Pts',(-1.30413842461196,225.476959054234,-7.38978847549663));
#12362=CARTESIAN_POINT('Ctrl Pts',(-1.15323012442366,225.411920847683,-7.41326423358633));
#12363=CARTESIAN_POINT('Ctrl Pts',(-1.00234807511957,225.346893954693,-7.43673590800797));
#12364=CARTESIAN_POINT('Ctrl Pts',(-0.850814170352588,225.281951283189,
-7.45558679680065));
#12365=CARTESIAN_POINT('Ctrl Pts',(-0.699053789843849,225.217273190525,
-7.46978916139897));
#12366=CARTESIAN_POINT('Ctrl Pts',(-0.547252685316753,225.152577741871,
-7.4839953371195));
#12367=CARTESIAN_POINT('Ctrl Pts',(-0.395225509158822,225.088147231022,
-7.49355053594383));
#12368=CARTESIAN_POINT('Ctrl Pts',(-0.243395891140422,225.02415727582,-7.49847882953767));
#12369=CARTESIAN_POINT('Ctrl Pts',(-0.225880023133874,225.016775056041,
-7.49904738356035));
#12370=CARTESIAN_POINT('Ctrl Pts',(-0.208366777074322,225.009398692253,
-7.49955441349819));
#12371=CARTESIAN_POINT('Ctrl Pts',(-0.19085679670529,225.002028447915,-7.5));
#12372=CARTESIAN_POINT('Ctrl Pts',(-0.0390720635510056,224.938139708658,
-7.50386255306115));
#12373=CARTESIAN_POINT('Ctrl Pts',(0.113193416374946,224.87379055128,-7.50312239555638));
#12374=CARTESIAN_POINT('Ctrl Pts',(0.265518780411738,224.809155844927,-7.49772806215971));
#12375=CARTESIAN_POINT('Ctrl Pts',(0.423677011228685,224.74204613624,-7.49212716810082));
#12376=CARTESIAN_POINT('Ctrl Pts',(0.581899244411136,224.674628800623,-7.48150838279936));
#12377=CARTESIAN_POINT('Ctrl Pts',(0.739708076930718,224.607105531561,-7.46587290795738));
#12378=CARTESIAN_POINT('Ctrl Pts',(0.891676432864649,224.542081286575,-7.4508160992348));
#12379=CARTESIAN_POINT('Ctrl Pts',(1.04326087688649,224.476959054234,-7.43110741988637));
#12380=CARTESIAN_POINT('Ctrl Pts',(1.19403760734915,224.411920847683,-7.40680096324213));
#12381=CARTESIAN_POINT('Ctrl Pts',(1.34478810981431,224.346893954693,-7.38249873476812));
#12382=CARTESIAN_POINT('Ctrl Pts',(1.49473066237841,224.281951283189,-7.35360044359541));
#12383=CARTESIAN_POINT('Ctrl Pts',(1.64345213319768,224.217273190526,-7.32021115834349));
#12384=CARTESIAN_POINT('Ctrl Pts',(1.79221351256174,224.152577741871,-7.28681291327038));
#12385=CARTESIAN_POINT('Ctrl Pts',(1.93975266792208,224.088147231022,-7.24892146633712));
#12386=CARTESIAN_POINT('Ctrl Pts',(2.08567414197888,224.02415727582,-7.20669061985661));
#12387=CARTESIAN_POINT('Ctrl Pts',(2.10250841524046,224.016775056041,-7.20181864597946));
#12388=CARTESIAN_POINT('Ctrl Pts',(2.11932118289448,224.009398692253,-7.19688896944667));
#12389=CARTESIAN_POINT('Ctrl Pts',(2.13611185762633,224.002028447915,-7.19190186588755));
#12390=CARTESIAN_POINT('Ctrl Pts',(2.28166131170461,223.938139708658,-7.14867131011448));
#12391=CARTESIAN_POINT('Ctrl Pts',(2.42624566734772,223.87379055128,-7.10091475754264));
#12392=CARTESIAN_POINT('Ctrl Pts',(2.56944875671925,223.809155844927,-7.04871331545287));
#12393=CARTESIAN_POINT('Ctrl Pts',(2.71813540129546,223.74204613624,-6.99451296753837));
#12394=CARTESIAN_POINT('Ctrl Pts',(2.86533230206858,223.674628800622,-6.93552054364095));
#12395=CARTESIAN_POINT('Ctrl Pts',(3.01058579312391,223.60710553156,-6.87188471229612));
#12396=CARTESIAN_POINT('Ctrl Pts',(3.1504634785292,223.542081286575,-6.81060403165508));
#12397=CARTESIAN_POINT('Ctrl Pts',(3.2885385349298,223.476959054234,-6.74501779444754));
#12398=CARTESIAN_POINT('Ctrl Pts',(3.42442461876589,223.411920847683,-6.67530840839872));
#12399=CARTESIAN_POINT('Ctrl Pts',(3.56028706487057,223.346893954693,-6.60561114847569));
#12400=CARTESIAN_POINT('Ctrl Pts',(3.69396084347589,223.281951283188,-6.53179244342376));
#12401=CARTESIAN_POINT('Ctrl Pts',(3.82508551083875,223.217273190525,-6.45407988419884));
#12402=CARTESIAN_POINT('Ctrl Pts',(3.95624536474612,223.152577741871,-6.37634647125905));
#12403=CARTESIAN_POINT('Ctrl Pts',(4.08485433881643,223.088147231022,-6.29471745739922));
#12404=CARTESIAN_POINT('Ctrl Pts',(4.21058385833625,223.024157275819,-6.20946132033745));
#12405=CARTESIAN_POINT('Ctrl Pts',(4.22508868089433,223.016775056041,-6.19962572130874));
#12406=CARTESIAN_POINT('Ctrl Pts',(4.239555219303,223.009398692253,-6.1897418893916));
#12407=CARTESIAN_POINT('Ctrl Pts',(4.253983000167,223.002028447915,-6.17981026821526));
#12408=CARTESIAN_POINT('Ctrl Pts',(4.379049780501,222.938139708658,-6.09371831161218));
#12409=CARTESIAN_POINT('Ctrl Pts',(4.50180008775205,222.87379055128,-6.00362010807862));
#12410=CARTESIAN_POINT('Ctrl Pts',(4.62186318631563,222.809155844927,-5.90972139815651));
#12411=CARTESIAN_POINT('Ctrl Pts',(4.74652375991935,222.74204613624,-5.81222710407629));
#12412=CARTESIAN_POINT('Ctrl Pts',(4.86828667005446,222.674628800623,-5.71063563105837));
#12413=CARTESIAN_POINT('Ctrl Pts',(4.98676639590057,222.607105531561,-5.60522856175958));
#12414=CARTESIAN_POINT('Ctrl Pts',(5.10086120834461,222.542081286575,-5.50372258918887));
#12415=CARTESIAN_POINT('Ctrl Pts',(5.21191112857799,222.476959054234,-5.39867883198631));
#12416=CARTESIAN_POINT('Ctrl Pts',(5.3196050891276,222.411920847683,-5.29039015693326));
#12417=CARTESIAN_POINT('Ctrl Pts',(5.42728031603795,222.346893954693,-5.18212031897158));
#12418=CARTESIAN_POINT('Ctrl Pts',(5.53160039987481,222.281951283188,-5.07060708921584));
#12419=CARTESIAN_POINT('Ctrl Pts',(5.63229286774066,222.217273190525,-4.95617830276981));
#12420=CARTESIAN_POINT('Ctrl Pts',(5.73301235584641,222.152577741871,-4.84171881002245));
#12421=CARTESIAN_POINT('Ctrl Pts',(5.83010200617326,222.088147231022,-4.72434264585545));
#12422=CARTESIAN_POINT('Ctrl Pts',(5.92333228977638,222.024157275819,-4.60440668292247));
#12423=CARTESIAN_POINT('Ctrl Pts',(5.93408782853811,222.016775056041,-4.59057023570385));
#12424=CARTESIAN_POINT('Ctrl Pts',(5.94479205212787,222.009398692253,-4.57669974673517));
#12425=CARTESIAN_POINT('Ctrl Pts',(5.95544464740896,222.002028447915,-4.56279578422009));
#12426=CARTESIAN_POINT('Ctrl Pts',(6.04778634614835,221.938139708658,-4.44226970733712));
#12427=CARTESIAN_POINT('Ctrl Pts',(6.13668694968221,221.87379055128,-4.31864929275467));
#12428=CARTESIAN_POINT('Ctrl Pts',(6.2218574448219,221.809155844927,-4.19224477495803));
#12429=CARTESIAN_POINT('Ctrl Pts',(6.31028930194743,221.74204613624,-4.06099995549937));
#12430=CARTESIAN_POINT('Ctrl Pts',(6.39469921942835,221.674628800622,-3.92675391456936));
#12431=CARTESIAN_POINT('Ctrl Pts',(6.47480755900257,221.607105531561,-3.78989358567385));
#12432=CARTESIAN_POINT('Ctrl Pts',(6.55195110329805,221.542081286575,-3.65809843300234));
#12433=CARTESIAN_POINT('Ctrl Pts',(6.62510554744149,221.476959054234,-3.5238795706426));
#12434=CARTESIAN_POINT('Ctrl Pts',(6.6940655494981,221.411920847683,-3.38761165659102));
#12435=CARTESIAN_POINT('Ctrl Pts',(6.76301355578647,221.346893954693,-3.25136744669064));
#12436=CARTESIAN_POINT('Ctrl Pts',(6.8277683682079,221.281951283188,-3.11307538411788));
#12437=CARTESIAN_POINT('Ctrl Pts',(6.88817215625612,221.217273190525,-2.9731314573403));
#12438=CARTESIAN_POINT('Ctrl Pts',(6.94859215331057,221.15257774187,-2.83314997742154));
#12439=CARTESIAN_POINT('Ctrl Pts',(7.00465866845661,221.088147231021,-2.69151625970376));
#12440=CARTESIAN_POINT('Ctrl Pts',(7.0562636864104,221.024157275819,-2.54864063859434));
#12441=CARTESIAN_POINT('Ctrl Pts',(7.06221711430353,221.016775056041,-2.53215775104408));
#12442=CARTESIAN_POINT('Ctrl Pts',(7.06811121908868,221.009398692253,-2.51565834512583));
#12443=CARTESIAN_POINT('Ctrl Pts',(7.07394587853975,221.002028447915,-2.4991430579979));
#12444=CARTESIAN_POINT('Ctrl Pts',(7.12452344682937,220.938139708658,-2.35598079299513));
#12445=CARTESIAN_POINT('Ctrl Pts',(7.17087213616511,220.87379055128,-2.21093899485743));
#12446=CARTESIAN_POINT('Ctrl Pts',(7.21281294639882,220.809155844927,-2.06440202410049));
#12447=CARTESIAN_POINT('Ctrl Pts',(7.25635976072976,220.74204613624,-1.91225383662838));
#12448=CARTESIAN_POINT('Ctrl Pts',(7.29515405471502,220.674628800623,-1.75849416561964));
#12449=CARTESIAN_POINT('Ctrl Pts',(7.32904944559223,220.607105531561,-1.60357741968163));
#12450=CARTESIAN_POINT('Ctrl Pts',(7.36169037413284,220.542081286575,-1.4543941147236));
#12451=CARTESIAN_POINT('Ctrl Pts',(7.38978847549659,220.476959054234,-1.30413842461222));
#12452=CARTESIAN_POINT('Ctrl Pts',(7.41326423358631,220.411920847683,-1.15323012442383));
#12453=CARTESIAN_POINT('Ctrl Pts',(7.43673590800786,220.346893954694,-1.00234807512029));
#12454=CARTESIAN_POINT('Ctrl Pts',(7.4555867968005,220.281951283189,-0.850814170353856));
#12455=CARTESIAN_POINT('Ctrl Pts',(7.4697891613988,220.217273190526,-0.69905378984567));
#12456=CARTESIAN_POINT('Ctrl Pts',(7.48399533711939,220.152577741872,-0.547252685318368));
#12457=CARTESIAN_POINT('Ctrl Pts',(7.49355053594376,220.088147231023,-0.395225509160228));
#12458=CARTESIAN_POINT('Ctrl Pts',(7.49847882953763,220.02415727582,-0.243395891141619));
#12459=CARTESIAN_POINT('Ctrl Pts',(7.49904738356033,220.016775056042,-0.22588002313467));
#12460=CARTESIAN_POINT('Ctrl Pts',(7.49955441349818,220.009398692253,-0.20836677707472));
#12461=CARTESIAN_POINT('Ctrl Pts',(7.5,220.002028447915,-0.190856796705287));
#12462=CARTESIAN_POINT('Ctrl Pts',(7.50386255306115,219.938139708658,-0.0390720635509813));
#12463=CARTESIAN_POINT('Ctrl Pts',(7.50312239555638,219.87379055128,0.113193416374992));
#12464=CARTESIAN_POINT('Ctrl Pts',(7.49772806215971,219.809155844927,0.265518780411804));
#12465=CARTESIAN_POINT('Ctrl Pts',(7.49212716810081,219.74204613624,0.423677011228746));
#12466=CARTESIAN_POINT('Ctrl Pts',(7.48150838279935,219.674628800622,0.581899244411192));
#12467=CARTESIAN_POINT('Ctrl Pts',(7.46587290795738,219.607105531561,0.739708076930769));
#12468=CARTESIAN_POINT('Ctrl Pts',(7.45081609923482,219.542081286575,0.891676432864501));
#12469=CARTESIAN_POINT('Ctrl Pts',(7.43110741988641,219.476959054234,1.04326087688616));
#12470=CARTESIAN_POINT('Ctrl Pts',(7.40680096324221,219.411920847683,1.19403760734863));
#12471=CARTESIAN_POINT('Ctrl Pts',(7.38249873476801,219.346893954693,1.34478810981507));
#12472=CARTESIAN_POINT('Ctrl Pts',(7.35360044359503,219.281951283188,1.49473066238045));
#12473=CARTESIAN_POINT('Ctrl Pts',(7.32021115834276,219.217273190524,1.64345213320097));
#12474=CARTESIAN_POINT('Ctrl Pts',(7.28681291326939,219.152577741869,1.79221351256585));
#12475=CARTESIAN_POINT('Ctrl Pts',(7.24892146633583,219.08814723102,1.93975266792699));
#12476=CARTESIAN_POINT('Ctrl Pts',(7.20669061985496,219.024157275817,2.08567414198458));
#12477=CARTESIAN_POINT('Ctrl Pts',(7.20181864597834,219.01677505604,2.10250841524425));
#12478=CARTESIAN_POINT('Ctrl Pts',(7.19688896944612,219.009398692252,2.11932118289636));
#12479=CARTESIAN_POINT('Ctrl Pts',(7.19190186588756,219.002028447915,2.13611185762631));
#12480=CARTESIAN_POINT('Ctrl Pts',(7.14867131011454,218.938139708658,2.28166131170442));
#12481=CARTESIAN_POINT('Ctrl Pts',(7.10091475754276,218.87379055128,2.42624566734735));
#12482=CARTESIAN_POINT('Ctrl Pts',(7.04871331545306,218.809155844927,2.56944875671871));
#12483=CARTESIAN_POINT('Ctrl Pts',(6.99451296753855,218.74204613624,2.71813540129498));
#12484=CARTESIAN_POINT('Ctrl Pts',(6.93552054364113,218.674628800622,2.86533230206815));
#12485=CARTESIAN_POINT('Ctrl Pts',(6.87188471229629,218.607105531561,3.01058579312352));
#12486=CARTESIAN_POINT('Ctrl Pts',(6.81060403165534,218.542081286575,3.15046347852863));
#12487=CARTESIAN_POINT('Ctrl Pts',(6.7450177944479,218.476959054234,3.28853853492905));
#12488=CARTESIAN_POINT('Ctrl Pts',(6.6753084083992,218.411920847683,3.42442461876496));
#12489=CARTESIAN_POINT('Ctrl Pts',(6.60561114847611,218.346893954694,3.56028706486978));
#12490=CARTESIAN_POINT('Ctrl Pts',(6.53179244342414,218.281951283189,3.69396084347523));
#12491=CARTESIAN_POINT('Ctrl Pts',(6.45407988419915,218.217273190526,3.82508551083821));
#12492=CARTESIAN_POINT('Ctrl Pts',(6.3763464712596,218.152577741871,3.95624536474522));
#12493=CARTESIAN_POINT('Ctrl Pts',(6.29471745740002,218.088147231023,4.0848543388152));
#12494=CARTESIAN_POINT('Ctrl Pts',(6.20946132033851,218.02415727582,4.21058385833468));
#12495=CARTESIAN_POINT('Ctrl Pts',(6.19962572130945,218.016775056042,4.22508868089329));
#12496=CARTESIAN_POINT('Ctrl Pts',(6.18974188939196,218.009398692253,4.23955521930249));
#12497=CARTESIAN_POINT('Ctrl Pts',(6.17981026821525,218.002028447915,4.25398300016701));
#12498=CARTESIAN_POINT('Ctrl Pts',(6.09371831161196,217.938139708658,4.37904978050132));
#12499=CARTESIAN_POINT('Ctrl Pts',(6.00362010807817,217.87379055128,4.50180008775267));
#12500=CARTESIAN_POINT('Ctrl Pts',(5.9097213981558,217.809155844927,4.62186318631654));
#12501=CARTESIAN_POINT('Ctrl Pts',(5.81222710407562,217.742046136239,4.74652375992017));
#12502=CARTESIAN_POINT('Ctrl Pts',(5.71063563105773,217.674628800622,4.8682866700552));
#12503=CARTESIAN_POINT('Ctrl Pts',(5.605228561759,217.60710553156,4.98676639590123));
#12504=CARTESIAN_POINT('Ctrl Pts',(5.50372258918827,217.542081286575,5.10086120834527));
#12505=CARTESIAN_POINT('Ctrl Pts',(5.3986788319857,217.476959054234,5.21191112857863));
#12506=CARTESIAN_POINT('Ctrl Pts',(5.29039015693262,217.411920847682,5.31960508912823));
#12507=CARTESIAN_POINT('Ctrl Pts',(5.18212031897114,217.346893954693,5.42728031603836));
#12508=CARTESIAN_POINT('Ctrl Pts',(5.07060708921561,217.281951283188,5.53160039987501));
#12509=CARTESIAN_POINT('Ctrl Pts',(4.95617830276981,217.217273190525,5.63229286774066));
#12510=CARTESIAN_POINT('Ctrl Pts',(4.84171881002289,217.152577741871,5.73301235584603));
#12511=CARTESIAN_POINT('Ctrl Pts',(4.72434264585635,217.088147231022,5.83010200617252));
#12512=CARTESIAN_POINT('Ctrl Pts',(4.60440668292385,217.02415727582,5.92333228977531));
#12513=CARTESIAN_POINT('Ctrl Pts',(4.59057023570477,217.016775056041,5.9340878285374));
#12514=CARTESIAN_POINT('Ctrl Pts',(4.57669974673563,217.009398692253,5.94479205212752));
#12515=CARTESIAN_POINT('Ctrl Pts',(4.56279578422008,217.002028447915,5.95544464740896));
#12516=CARTESIAN_POINT('Ctrl Pts',(4.44226970733684,216.938139708657,6.04778634614857));
#12517=CARTESIAN_POINT('Ctrl Pts',(4.31864929275411,216.87379055128,6.13668694968261));
#12518=CARTESIAN_POINT('Ctrl Pts',(4.19224477495716,216.809155844927,6.22185744482248));
#12519=CARTESIAN_POINT('Ctrl Pts',(4.06099995549857,216.742046136239,6.31028930194794));
#12520=CARTESIAN_POINT('Ctrl Pts',(3.92675391456862,216.674628800622,6.3946992194288));
#12521=CARTESIAN_POINT('Ctrl Pts',(3.78989358567318,216.60710553156,6.47480755900296));
#12522=CARTESIAN_POINT('Ctrl Pts',(3.65809843300166,216.542081286575,6.55195110329844));
#12523=CARTESIAN_POINT('Ctrl Pts',(3.5238795706419,216.476959054234,6.62510554744185));
#12524=CARTESIAN_POINT('Ctrl Pts',(3.38761165659031,216.411920847682,6.69406554949845));
#12525=CARTESIAN_POINT('Ctrl Pts',(3.25136744669046,216.346893954693,6.76301355578654));
#12526=CARTESIAN_POINT('Ctrl Pts',(3.11307538411824,216.281951283188,6.82776836820773));
#12527=CARTESIAN_POINT('Ctrl Pts',(2.97313145734122,216.217273190525,6.88817215625573));
#12528=CARTESIAN_POINT('Ctrl Pts',(2.83314997742261,216.152577741871,6.94859215331013));
#12529=CARTESIAN_POINT('Ctrl Pts',(2.69151625970498,216.088147231022,7.00465866845613));
#12530=CARTESIAN_POINT('Ctrl Pts',(2.54864063859571,216.024157275819,7.0562636864099));
#12531=CARTESIAN_POINT('Ctrl Pts',(2.532157751045,216.016775056041,7.0622171143032));
#12532=CARTESIAN_POINT('Ctrl Pts',(2.51565834512628,216.009398692253,7.06811121908852));
#12533=CARTESIAN_POINT('Ctrl Pts',(2.49914305799789,216.002028447915,7.07394587853975));
#12534=CARTESIAN_POINT('Ctrl Pts',(2.35598079299496,215.938139708658,7.12452344682943));
#12535=CARTESIAN_POINT('Ctrl Pts',(2.2109389948571,215.87379055128,7.17087213616521));
#12536=CARTESIAN_POINT('Ctrl Pts',(2.0644020241,215.809155844927,7.21281294639896));
#12537=CARTESIAN_POINT('Ctrl Pts',(1.91225383662793,215.74204613624,7.25635976072988));
#12538=CARTESIAN_POINT('Ctrl Pts',(1.75849416561922,215.674628800623,7.29515405471512));
#12539=CARTESIAN_POINT('Ctrl Pts',(1.60357741968125,215.607105531561,7.32904944559231));
#12540=CARTESIAN_POINT('Ctrl Pts',(1.4543941147233,215.542081286575,7.3616903741329));
#12541=CARTESIAN_POINT('Ctrl Pts',(1.30413842461201,215.476959054234,7.38978847549662));
#12542=CARTESIAN_POINT('Ctrl Pts',(1.15323012442371,215.411920847683,7.41326423358633));
#12543=CARTESIAN_POINT('Ctrl Pts',(1.00234807511962,215.346893954693,7.43673590800796));
#12544=CARTESIAN_POINT('Ctrl Pts',(0.85081417035265,215.281951283189,7.45558679680064));
#12545=CARTESIAN_POINT('Ctrl Pts',(0.699053789843915,215.217273190525,7.46978916139897));
#12546=CARTESIAN_POINT('Ctrl Pts',(0.547252685316762,215.152577741871,7.4839953371195));
#12547=CARTESIAN_POINT('Ctrl Pts',(0.395225509158773,215.088147231022,7.49355053594384));
#12548=CARTESIAN_POINT('Ctrl Pts',(0.243395891140316,215.02415727582,7.49847882953767));
#12549=CARTESIAN_POINT('Ctrl Pts',(0.225880023133805,215.016775056041,7.49904738356035));
#12550=CARTESIAN_POINT('Ctrl Pts',(0.208366777074288,215.009398692253,7.49955441349819));
#12551=CARTESIAN_POINT('Ctrl Pts',(0.190856796705293,215.002028447915,7.5));
#12552=CARTESIAN_POINT('Ctrl Pts',(0.127311648028422,214.975281229334,7.50161706980302));
#12553=CARTESIAN_POINT('Ctrl Pts',(0.0636823578853861,214.948453397593,
7.50242803155527));
#12554=CARTESIAN_POINT('Ctrl Pts',(-4.068439266928E-7,214.921557632927,
7.50242802810187));
#12555=CARTESIAN_POINT('Origin',(0.,240.,0.));
#12556=CARTESIAN_POINT('Origin',(0.190856796705285,235.002028447915,28.7581985010212));
#12557=CARTESIAN_POINT('',(0.190856796705285,235.002028447915,50.0163970020424));
#12558=CARTESIAN_POINT('Ctrl Pts',(0.190856796705285,235.002028447915,7.5));
#12559=CARTESIAN_POINT('Ctrl Pts',(0.190856796705285,235.002028447915,14.5858638315753));
#12560=CARTESIAN_POINT('Ctrl Pts',(0.190856796705285,235.002028447915,21.6717276631507));
#12561=CARTESIAN_POINT('Ctrl Pts',(0.190856796705285,235.002028447915,35.8438599971648));
#12562=CARTESIAN_POINT('Ctrl Pts',(0.190856796705285,235.002028447915,42.9301284996036));
#12563=CARTESIAN_POINT('Ctrl Pts',(0.190856796705285,235.002028447915,50.0163970020424));
#12564=CARTESIAN_POINT('',(0.000256710972400845,237.995967593475,50.0163970020424));
#12565=CARTESIAN_POINT('',(0.000256710972400879,237.995967593475,50.0163970020424));
#12566=CARTESIAN_POINT('',(0.190856796705286,235.002028447915,50.0163970020424));
#12567=CARTESIAN_POINT('Origin',(0.190856796705285,175.002028447915,28.7581985010212));
#12568=CARTESIAN_POINT('',(0.190856796705285,175.002028447915,50.0163970020424));
#12569=CARTESIAN_POINT('Ctrl Pts',(0.190856796705285,175.002028447915,50.0163970020424));
#12570=CARTESIAN_POINT('Ctrl Pts',(0.190856796705285,175.002028447915,42.9301284996036));
#12571=CARTESIAN_POINT('Ctrl Pts',(0.190856796705285,175.002028447915,35.8438599971648));
#12572=CARTESIAN_POINT('Ctrl Pts',(0.190856796705285,175.002028447915,21.6717276631507));
#12573=CARTESIAN_POINT('Ctrl Pts',(0.190856796705285,175.002028447915,14.5858638315753));
#12574=CARTESIAN_POINT('Ctrl Pts',(0.190856796705285,175.002028447915,7.5));
#12575=CARTESIAN_POINT('',(0.000256710972400845,177.995967593475,50.0163970020424));
#12576=CARTESIAN_POINT('',(0.000256710972401712,177.995967593475,50.0163970020424));
#12577=CARTESIAN_POINT('',(0.00025671097240121,177.995967593475,7.5));
#12578=CARTESIAN_POINT('Ctrl Pts',(0.190856796705285,235.002028447915,7.5));
#12579=CARTESIAN_POINT('Ctrl Pts',(-0.997026505728737,234.502028447915,
7.5302287469283));
#12580=CARTESIAN_POINT('Ctrl Pts',(-2.13611185762632,234.002028447915,7.19190186588755));
#12581=CARTESIAN_POINT('Ctrl Pts',(-3.27519720952391,233.502028447915,6.8535749848468));
#12582=CARTESIAN_POINT('Ctrl Pts',(-4.25398300016701,233.002028447915,6.17981026821526));
#12583=CARTESIAN_POINT('Ctrl Pts',(-5.2327687908101,232.502028447915,5.50604555158371));
#12584=CARTESIAN_POINT('Ctrl Pts',(-5.95544464740896,232.002028447915,4.56279578422009));
#12585=CARTESIAN_POINT('Ctrl Pts',(-6.67812050400781,231.502028447915,3.61954601685647));
#12586=CARTESIAN_POINT('Ctrl Pts',(-7.07394587853975,231.002028447915,2.49914305799789));
#12587=CARTESIAN_POINT('Ctrl Pts',(-7.4697712530717,230.502028447915,1.37874009913931));
#12588=CARTESIAN_POINT('Ctrl Pts',(-7.5,230.002028447915,0.190856796705286));
#12589=CARTESIAN_POINT('Ctrl Pts',(-7.5302287469283,229.502028447915,-0.997026505728736));
#12590=CARTESIAN_POINT('Ctrl Pts',(-7.19190186588755,229.002028447915,-2.13611185762632));
#12591=CARTESIAN_POINT('Ctrl Pts',(-6.8535749848468,228.502028447915,-3.27519720952391));
#12592=CARTESIAN_POINT('Ctrl Pts',(-6.17981026821526,228.002028447915,-4.25398300016701));
#12593=CARTESIAN_POINT('Ctrl Pts',(-5.50604555158371,227.502028447915,-5.2327687908101));
#12594=CARTESIAN_POINT('Ctrl Pts',(-4.56279578422009,227.002028447915,-5.95544464740895));
#12595=CARTESIAN_POINT('Ctrl Pts',(-3.61954601685647,226.502028447915,-6.67812050400781));
#12596=CARTESIAN_POINT('Ctrl Pts',(-2.49914305799789,226.002028447915,-7.07394587853975));
#12597=CARTESIAN_POINT('Ctrl Pts',(-1.37874009913931,225.502028447915,-7.4697712530717));
#12598=CARTESIAN_POINT('Ctrl Pts',(-0.190856796705286,225.002028447915,
-7.5));
#12599=CARTESIAN_POINT('Ctrl Pts',(0.997026505728736,224.502028447915,-7.5302287469283));
#12600=CARTESIAN_POINT('Ctrl Pts',(2.13611185762632,224.002028447915,-7.19190186588755));
#12601=CARTESIAN_POINT('Ctrl Pts',(3.27519720952391,223.502028447915,-6.8535749848468));
#12602=CARTESIAN_POINT('Ctrl Pts',(4.25398300016701,223.002028447915,-6.17981026821526));
#12603=CARTESIAN_POINT('Ctrl Pts',(5.2327687908101,222.502028447915,-5.50604555158371));
#12604=CARTESIAN_POINT('Ctrl Pts',(5.95544464740895,222.002028447915,-4.56279578422009));
#12605=CARTESIAN_POINT('Ctrl Pts',(6.67812050400781,221.502028447915,-3.61954601685647));
#12606=CARTESIAN_POINT('Ctrl Pts',(7.07394587853975,221.002028447915,-2.49914305799789));
#12607=CARTESIAN_POINT('Ctrl Pts',(7.4697712530717,220.502028447915,-1.37874009913931));
#12608=CARTESIAN_POINT('Ctrl Pts',(7.5,220.002028447915,-0.190856796705287));
#12609=CARTESIAN_POINT('Ctrl Pts',(7.5302287469283,219.502028447915,0.997026505728735));
#12610=CARTESIAN_POINT('Ctrl Pts',(7.19190186588755,219.002028447915,2.13611185762632));
#12611=CARTESIAN_POINT('Ctrl Pts',(6.8535749848468,218.502028447915,3.27519720952391));
#12612=CARTESIAN_POINT('Ctrl Pts',(6.17981026821526,218.002028447915,4.25398300016701));
#12613=CARTESIAN_POINT('Ctrl Pts',(5.50604555158371,217.502028447915,5.2327687908101));
#12614=CARTESIAN_POINT('Ctrl Pts',(4.56279578422009,217.002028447915,5.95544464740895));
#12615=CARTESIAN_POINT('Ctrl Pts',(3.61954601685647,216.502028447915,6.67812050400781));
#12616=CARTESIAN_POINT('Ctrl Pts',(2.49914305799789,216.002028447915,7.07394587853975));
#12617=CARTESIAN_POINT('Ctrl Pts',(1.37874009913931,215.502028447915,7.4697712530717));
#12618=CARTESIAN_POINT('Ctrl Pts',(0.190856796705285,215.002028447915,7.5));
#12619=CARTESIAN_POINT('Ctrl Pts',(-0.997026505728737,214.502028447915,
7.5302287469283));
#12620=CARTESIAN_POINT('Ctrl Pts',(-2.13611185762632,214.002028447915,7.19190186588755));
#12621=CARTESIAN_POINT('Ctrl Pts',(-3.27519720952391,213.502028447915,6.8535749848468));
#12622=CARTESIAN_POINT('Ctrl Pts',(-4.25398300016701,213.002028447915,6.17981026821526));
#12623=CARTESIAN_POINT('Ctrl Pts',(-5.2327687908101,212.502028447915,5.50604555158371));
#12624=CARTESIAN_POINT('Ctrl Pts',(-5.95544464740896,212.002028447915,4.56279578422009));
#12625=CARTESIAN_POINT('Ctrl Pts',(-6.67812050400781,211.502028447915,3.61954601685647));
#12626=CARTESIAN_POINT('Ctrl Pts',(-7.07394587853975,211.002028447915,2.49914305799789));
#12627=CARTESIAN_POINT('Ctrl Pts',(-7.4697712530717,210.502028447915,1.37874009913931));
#12628=CARTESIAN_POINT('Ctrl Pts',(-7.5,210.002028447915,0.190856796705286));
#12629=CARTESIAN_POINT('Ctrl Pts',(-7.5302287469283,209.502028447915,-0.997026505728736));
#12630=CARTESIAN_POINT('Ctrl Pts',(-7.19190186588755,209.002028447915,-2.13611185762632));
#12631=CARTESIAN_POINT('Ctrl Pts',(-6.8535749848468,208.502028447915,-3.27519720952391));
#12632=CARTESIAN_POINT('Ctrl Pts',(-6.17981026821526,208.002028447915,-4.25398300016701));
#12633=CARTESIAN_POINT('Ctrl Pts',(-5.50604555158371,207.502028447915,-5.2327687908101));
#12634=CARTESIAN_POINT('Ctrl Pts',(-4.56279578422009,207.002028447915,-5.95544464740895));
#12635=CARTESIAN_POINT('Ctrl Pts',(-3.61954601685647,206.502028447915,-6.67812050400781));
#12636=CARTESIAN_POINT('Ctrl Pts',(-2.49914305799789,206.002028447915,-7.07394587853975));
#12637=CARTESIAN_POINT('Ctrl Pts',(-1.37874009913931,205.502028447915,-7.4697712530717));
#12638=CARTESIAN_POINT('Ctrl Pts',(-0.190856796705286,205.002028447915,
-7.5));
#12639=CARTESIAN_POINT('Ctrl Pts',(0.997026505728736,204.502028447915,-7.5302287469283));
#12640=CARTESIAN_POINT('Ctrl Pts',(2.13611185762632,204.002028447915,-7.19190186588755));
#12641=CARTESIAN_POINT('Ctrl Pts',(3.27519720952391,203.502028447915,-6.8535749848468));
#12642=CARTESIAN_POINT('Ctrl Pts',(4.25398300016701,203.002028447915,-6.17981026821526));
#12643=CARTESIAN_POINT('Ctrl Pts',(5.2327687908101,202.502028447915,-5.50604555158371));
#12644=CARTESIAN_POINT('Ctrl Pts',(5.95544464740895,202.002028447915,-4.56279578422009));
#12645=CARTESIAN_POINT('Ctrl Pts',(6.67812050400781,201.502028447915,-3.61954601685647));
#12646=CARTESIAN_POINT('Ctrl Pts',(7.07394587853975,201.002028447915,-2.49914305799789));
#12647=CARTESIAN_POINT('Ctrl Pts',(7.4697712530717,200.502028447915,-1.37874009913931));
#12648=CARTESIAN_POINT('Ctrl Pts',(7.5,200.002028447915,-0.190856796705287));
#12649=CARTESIAN_POINT('Ctrl Pts',(7.5302287469283,199.502028447915,0.997026505728735));
#12650=CARTESIAN_POINT('Ctrl Pts',(7.19190186588755,199.002028447915,2.13611185762632));
#12651=CARTESIAN_POINT('Ctrl Pts',(6.8535749848468,198.502028447915,3.27519720952391));
#12652=CARTESIAN_POINT('Ctrl Pts',(6.17981026821526,198.002028447915,4.25398300016701));
#12653=CARTESIAN_POINT('Ctrl Pts',(5.50604555158371,197.502028447915,5.2327687908101));
#12654=CARTESIAN_POINT('Ctrl Pts',(4.56279578422009,197.002028447915,5.95544464740895));
#12655=CARTESIAN_POINT('Ctrl Pts',(3.61954601685647,196.502028447915,6.67812050400781));
#12656=CARTESIAN_POINT('Ctrl Pts',(2.49914305799789,196.002028447915,7.07394587853975));
#12657=CARTESIAN_POINT('Ctrl Pts',(1.37874009913931,195.502028447915,7.4697712530717));
#12658=CARTESIAN_POINT('Ctrl Pts',(0.190856796705285,195.002028447915,7.5));
#12659=CARTESIAN_POINT('Ctrl Pts',(-0.997026505728737,194.502028447915,
7.5302287469283));
#12660=CARTESIAN_POINT('Ctrl Pts',(-2.13611185762632,194.002028447915,7.19190186588755));
#12661=CARTESIAN_POINT('Ctrl Pts',(-3.27519720952391,193.502028447915,6.8535749848468));
#12662=CARTESIAN_POINT('Ctrl Pts',(-4.25398300016701,193.002028447915,6.17981026821526));
#12663=CARTESIAN_POINT('Ctrl Pts',(-5.2327687908101,192.502028447915,5.50604555158371));
#12664=CARTESIAN_POINT('Ctrl Pts',(-5.95544464740896,192.002028447915,4.56279578422009));
#12665=CARTESIAN_POINT('Ctrl Pts',(-6.67812050400781,191.502028447915,3.61954601685647));
#12666=CARTESIAN_POINT('Ctrl Pts',(-7.07394587853975,191.002028447915,2.49914305799789));
#12667=CARTESIAN_POINT('Ctrl Pts',(-7.4697712530717,190.502028447915,1.37874009913931));
#12668=CARTESIAN_POINT('Ctrl Pts',(-7.5,190.002028447915,0.190856796705286));
#12669=CARTESIAN_POINT('Ctrl Pts',(-7.5302287469283,189.502028447915,-0.997026505728736));
#12670=CARTESIAN_POINT('Ctrl Pts',(-7.19190186588755,189.002028447915,-2.13611185762632));
#12671=CARTESIAN_POINT('Ctrl Pts',(-6.8535749848468,188.502028447915,-3.27519720952391));
#12672=CARTESIAN_POINT('Ctrl Pts',(-6.17981026821526,188.002028447915,-4.25398300016701));
#12673=CARTESIAN_POINT('Ctrl Pts',(-5.50604555158371,187.502028447915,-5.2327687908101));
#12674=CARTESIAN_POINT('Ctrl Pts',(-4.56279578422009,187.002028447915,-5.95544464740895));
#12675=CARTESIAN_POINT('Ctrl Pts',(-3.61954601685647,186.502028447915,-6.67812050400781));
#12676=CARTESIAN_POINT('Ctrl Pts',(-2.49914305799789,186.002028447915,-7.07394587853975));
#12677=CARTESIAN_POINT('Ctrl Pts',(-1.37874009913931,185.502028447915,-7.4697712530717));
#12678=CARTESIAN_POINT('Ctrl Pts',(-0.190856796705286,185.002028447915,
-7.5));
#12679=CARTESIAN_POINT('Ctrl Pts',(0.997026505728736,184.502028447915,-7.5302287469283));
#12680=CARTESIAN_POINT('Ctrl Pts',(2.13611185762632,184.002028447915,-7.19190186588755));
#12681=CARTESIAN_POINT('Ctrl Pts',(3.27519720952391,183.502028447915,-6.8535749848468));
#12682=CARTESIAN_POINT('Ctrl Pts',(4.25398300016701,183.002028447915,-6.17981026821526));
#12683=CARTESIAN_POINT('Ctrl Pts',(5.2327687908101,182.502028447915,-5.50604555158371));
#12684=CARTESIAN_POINT('Ctrl Pts',(5.95544464740895,182.002028447915,-4.56279578422009));
#12685=CARTESIAN_POINT('Ctrl Pts',(6.67812050400781,181.502028447915,-3.61954601685647));
#12686=CARTESIAN_POINT('Ctrl Pts',(7.07394587853975,181.002028447915,-2.49914305799789));
#12687=CARTESIAN_POINT('Ctrl Pts',(7.4697712530717,180.502028447915,-1.37874009913931));
#12688=CARTESIAN_POINT('Ctrl Pts',(7.5,180.002028447915,-0.190856796705287));
#12689=CARTESIAN_POINT('Ctrl Pts',(7.5302287469283,179.502028447915,0.997026505728735));
#12690=CARTESIAN_POINT('Ctrl Pts',(7.19190186588755,179.002028447915,2.13611185762632));
#12691=CARTESIAN_POINT('Ctrl Pts',(6.8535749848468,178.502028447915,3.27519720952391));
#12692=CARTESIAN_POINT('Ctrl Pts',(6.17981026821526,178.002028447915,4.25398300016701));
#12693=CARTESIAN_POINT('Ctrl Pts',(5.50604555158371,177.502028447915,5.2327687908101));
#12694=CARTESIAN_POINT('Ctrl Pts',(4.56279578422009,177.002028447915,5.95544464740895));
#12695=CARTESIAN_POINT('Ctrl Pts',(3.61954601685647,176.502028447915,6.67812050400781));
#12696=CARTESIAN_POINT('Ctrl Pts',(2.49914305799789,176.002028447915,7.07394587853975));
#12697=CARTESIAN_POINT('Ctrl Pts',(1.37874009913931,175.502028447915,7.4697712530717));
#12698=CARTESIAN_POINT('Ctrl Pts',(0.190856796705285,175.002028447915,7.5));
#12699=CARTESIAN_POINT('Ctrl Pts',(0.190856796705285,235.002028447915,50.0163970020424));
#12700=CARTESIAN_POINT('Ctrl Pts',(-7.73096224951301,234.502028447915,50.0466257489707));
#12701=CARTESIAN_POINT('Ctrl Pts',(-15.2744010708495,234.002028447915,47.6273982840717));
#12702=CARTESIAN_POINT('Ctrl Pts',(-22.817839892186,233.502028447915,45.2081708191727));
#12703=CARTESIAN_POINT('Ctrl Pts',(-29.2444941385794,233.002028447915,40.5762979824596));
#12704=CARTESIAN_POINT('Ctrl Pts',(-35.6711483849729,232.502028447915,35.9444251457465));
#12705=CARTESIAN_POINT('Ctrl Pts',(-40.3519323616533,232.002028447915,29.5533069226325));
#12706=CARTESIAN_POINT('Ctrl Pts',(-45.0327163383337,231.502028447915,23.1621886995185));
#12707=CARTESIAN_POINT('Ctrl Pts',(-47.5094422967239,231.002028447915,15.6374322712211));
#12708=CARTESIAN_POINT('Ctrl Pts',(-49.9861682551141,230.502028447915,8.11267584292358));
#12709=CARTESIAN_POINT('Ctrl Pts',(-50.0163970020424,230.002028447915,0.190856796705288));
#12710=CARTESIAN_POINT('Ctrl Pts',(-50.0466257489707,229.502028447915,-7.73096224951301));
#12711=CARTESIAN_POINT('Ctrl Pts',(-47.6273982840717,229.002028447915,-15.2744010708495));
#12712=CARTESIAN_POINT('Ctrl Pts',(-45.2081708191727,228.502028447915,-22.817839892186));
#12713=CARTESIAN_POINT('Ctrl Pts',(-40.5762979824596,228.002028447915,-29.2444941385794));
#12714=CARTESIAN_POINT('Ctrl Pts',(-35.9444251457465,227.502028447915,-35.6711483849729));
#12715=CARTESIAN_POINT('Ctrl Pts',(-29.5533069226325,227.002028447915,-40.3519323616533));
#12716=CARTESIAN_POINT('Ctrl Pts',(-23.1621886995185,226.502028447915,-45.0327163383337));
#12717=CARTESIAN_POINT('Ctrl Pts',(-15.6374322712211,226.002028447915,-47.5094422967239));
#12718=CARTESIAN_POINT('Ctrl Pts',(-8.11267584292359,225.502028447915,-49.9861682551141));
#12719=CARTESIAN_POINT('Ctrl Pts',(-0.190856796705292,225.002028447915,
-50.0163970020424));
#12720=CARTESIAN_POINT('Ctrl Pts',(7.730962249513,224.502028447915,-50.0466257489707));
#12721=CARTESIAN_POINT('Ctrl Pts',(15.2744010708495,224.002028447915,-47.6273982840717));
#12722=CARTESIAN_POINT('Ctrl Pts',(22.817839892186,223.502028447915,-45.2081708191727));
#12723=CARTESIAN_POINT('Ctrl Pts',(29.2444941385794,223.002028447915,-40.5762979824596));
#12724=CARTESIAN_POINT('Ctrl Pts',(35.6711483849729,222.502028447915,-35.9444251457465));
#12725=CARTESIAN_POINT('Ctrl Pts',(40.3519323616533,222.002028447915,-29.5533069226325));
#12726=CARTESIAN_POINT('Ctrl Pts',(45.0327163383337,221.502028447915,-23.1621886995185));
#12727=CARTESIAN_POINT('Ctrl Pts',(47.5094422967239,221.002028447915,-15.6374322712211));
#12728=CARTESIAN_POINT('Ctrl Pts',(49.9861682551141,220.502028447915,-8.11267584292359));
#12729=CARTESIAN_POINT('Ctrl Pts',(50.0163970020424,220.002028447915,-0.190856796705295));
#12730=CARTESIAN_POINT('Ctrl Pts',(50.0466257489707,219.502028447915,7.730962249513));
#12731=CARTESIAN_POINT('Ctrl Pts',(47.6273982840717,219.002028447915,15.2744010708495));
#12732=CARTESIAN_POINT('Ctrl Pts',(45.2081708191727,218.502028447915,22.817839892186));
#12733=CARTESIAN_POINT('Ctrl Pts',(40.5762979824596,218.002028447915,29.2444941385794));
#12734=CARTESIAN_POINT('Ctrl Pts',(35.9444251457465,217.502028447915,35.6711483849729));
#12735=CARTESIAN_POINT('Ctrl Pts',(29.5533069226325,217.002028447915,40.3519323616533));
#12736=CARTESIAN_POINT('Ctrl Pts',(23.1621886995185,216.502028447915,45.0327163383337));
#12737=CARTESIAN_POINT('Ctrl Pts',(15.6374322712211,216.002028447915,47.5094422967239));
#12738=CARTESIAN_POINT('Ctrl Pts',(8.11267584292359,215.502028447915,49.9861682551141));
#12739=CARTESIAN_POINT('Ctrl Pts',(0.190856796705285,215.002028447915,50.0163970020424));
#12740=CARTESIAN_POINT('Ctrl Pts',(-7.73096224951301,214.502028447915,50.0466257489707));
#12741=CARTESIAN_POINT('Ctrl Pts',(-15.2744010708495,214.002028447915,47.6273982840717));
#12742=CARTESIAN_POINT('Ctrl Pts',(-22.817839892186,213.502028447915,45.2081708191727));
#12743=CARTESIAN_POINT('Ctrl Pts',(-29.2444941385794,213.002028447915,40.5762979824596));
#12744=CARTESIAN_POINT('Ctrl Pts',(-35.6711483849729,212.502028447915,35.9444251457465));
#12745=CARTESIAN_POINT('Ctrl Pts',(-40.3519323616533,212.002028447915,29.5533069226325));
#12746=CARTESIAN_POINT('Ctrl Pts',(-45.0327163383337,211.502028447915,23.1621886995185));
#12747=CARTESIAN_POINT('Ctrl Pts',(-47.5094422967239,211.002028447915,15.6374322712211));
#12748=CARTESIAN_POINT('Ctrl Pts',(-49.9861682551141,210.502028447915,8.11267584292358));
#12749=CARTESIAN_POINT('Ctrl Pts',(-50.0163970020424,210.002028447915,0.190856796705288));
#12750=CARTESIAN_POINT('Ctrl Pts',(-50.0466257489707,209.502028447915,-7.73096224951301));
#12751=CARTESIAN_POINT('Ctrl Pts',(-47.6273982840717,209.002028447915,-15.2744010708495));
#12752=CARTESIAN_POINT('Ctrl Pts',(-45.2081708191727,208.502028447915,-22.817839892186));
#12753=CARTESIAN_POINT('Ctrl Pts',(-40.5762979824596,208.002028447915,-29.2444941385794));
#12754=CARTESIAN_POINT('Ctrl Pts',(-35.9444251457465,207.502028447915,-35.6711483849729));
#12755=CARTESIAN_POINT('Ctrl Pts',(-29.5533069226325,207.002028447915,-40.3519323616533));
#12756=CARTESIAN_POINT('Ctrl Pts',(-23.1621886995185,206.502028447915,-45.0327163383337));
#12757=CARTESIAN_POINT('Ctrl Pts',(-15.6374322712211,206.002028447915,-47.5094422967239));
#12758=CARTESIAN_POINT('Ctrl Pts',(-8.11267584292359,205.502028447915,-49.9861682551141));
#12759=CARTESIAN_POINT('Ctrl Pts',(-0.190856796705292,205.002028447915,
-50.0163970020424));
#12760=CARTESIAN_POINT('Ctrl Pts',(7.730962249513,204.502028447915,-50.0466257489707));
#12761=CARTESIAN_POINT('Ctrl Pts',(15.2744010708495,204.002028447915,-47.6273982840717));
#12762=CARTESIAN_POINT('Ctrl Pts',(22.817839892186,203.502028447915,-45.2081708191727));
#12763=CARTESIAN_POINT('Ctrl Pts',(29.2444941385794,203.002028447915,-40.5762979824596));
#12764=CARTESIAN_POINT('Ctrl Pts',(35.6711483849729,202.502028447915,-35.9444251457465));
#12765=CARTESIAN_POINT('Ctrl Pts',(40.3519323616533,202.002028447915,-29.5533069226325));
#12766=CARTESIAN_POINT('Ctrl Pts',(45.0327163383337,201.502028447915,-23.1621886995185));
#12767=CARTESIAN_POINT('Ctrl Pts',(47.5094422967239,201.002028447915,-15.6374322712211));
#12768=CARTESIAN_POINT('Ctrl Pts',(49.9861682551141,200.502028447915,-8.11267584292359));
#12769=CARTESIAN_POINT('Ctrl Pts',(50.0163970020424,200.002028447915,-0.190856796705295));
#12770=CARTESIAN_POINT('Ctrl Pts',(50.0466257489707,199.502028447915,7.730962249513));
#12771=CARTESIAN_POINT('Ctrl Pts',(47.6273982840717,199.002028447915,15.2744010708495));
#12772=CARTESIAN_POINT('Ctrl Pts',(45.2081708191727,198.502028447915,22.817839892186));
#12773=CARTESIAN_POINT('Ctrl Pts',(40.5762979824596,198.002028447915,29.2444941385794));
#12774=CARTESIAN_POINT('Ctrl Pts',(35.9444251457465,197.502028447915,35.6711483849729));
#12775=CARTESIAN_POINT('Ctrl Pts',(29.5533069226325,197.002028447915,40.3519323616533));
#12776=CARTESIAN_POINT('Ctrl Pts',(23.1621886995185,196.502028447915,45.0327163383337));
#12777=CARTESIAN_POINT('Ctrl Pts',(15.6374322712211,196.002028447915,47.5094422967239));
#12778=CARTESIAN_POINT('Ctrl Pts',(8.11267584292359,195.502028447915,49.9861682551141));
#12779=CARTESIAN_POINT('Ctrl Pts',(0.190856796705285,195.002028447915,50.0163970020424));
#12780=CARTESIAN_POINT('Ctrl Pts',(-7.73096224951301,194.502028447915,50.0466257489707));
#12781=CARTESIAN_POINT('Ctrl Pts',(-15.2744010708495,194.002028447915,47.6273982840717));
#12782=CARTESIAN_POINT('Ctrl Pts',(-22.817839892186,193.502028447915,45.2081708191727));
#12783=CARTESIAN_POINT('Ctrl Pts',(-29.2444941385794,193.002028447915,40.5762979824596));
#12784=CARTESIAN_POINT('Ctrl Pts',(-35.6711483849729,192.502028447915,35.9444251457465));
#12785=CARTESIAN_POINT('Ctrl Pts',(-40.3519323616533,192.002028447915,29.5533069226325));
#12786=CARTESIAN_POINT('Ctrl Pts',(-45.0327163383337,191.502028447915,23.1621886995185));
#12787=CARTESIAN_POINT('Ctrl Pts',(-47.5094422967239,191.002028447915,15.6374322712211));
#12788=CARTESIAN_POINT('Ctrl Pts',(-49.9861682551141,190.502028447915,8.11267584292358));
#12789=CARTESIAN_POINT('Ctrl Pts',(-50.0163970020424,190.002028447915,0.190856796705288));
#12790=CARTESIAN_POINT('Ctrl Pts',(-50.0466257489707,189.502028447915,-7.73096224951301));
#12791=CARTESIAN_POINT('Ctrl Pts',(-47.6273982840717,189.002028447915,-15.2744010708495));
#12792=CARTESIAN_POINT('Ctrl Pts',(-45.2081708191727,188.502028447915,-22.817839892186));
#12793=CARTESIAN_POINT('Ctrl Pts',(-40.5762979824596,188.002028447915,-29.2444941385794));
#12794=CARTESIAN_POINT('Ctrl Pts',(-35.9444251457465,187.502028447915,-35.6711483849729));
#12795=CARTESIAN_POINT('Ctrl Pts',(-29.5533069226325,187.002028447915,-40.3519323616533));
#12796=CARTESIAN_POINT('Ctrl Pts',(-23.1621886995185,186.502028447915,-45.0327163383337));
#12797=CARTESIAN_POINT('Ctrl Pts',(-15.6374322712211,186.002028447915,-47.5094422967239));
#12798=CARTESIAN_POINT('Ctrl Pts',(-8.11267584292359,185.502028447915,-49.9861682551141));
#12799=CARTESIAN_POINT('Ctrl Pts',(-0.190856796705292,185.002028447915,
-50.0163970020424));
#12800=CARTESIAN_POINT('Ctrl Pts',(7.730962249513,184.502028447915,-50.0466257489707));
#12801=CARTESIAN_POINT('Ctrl Pts',(15.2744010708495,184.002028447915,-47.6273982840717));
#12802=CARTESIAN_POINT('Ctrl Pts',(22.817839892186,183.502028447915,-45.2081708191727));
#12803=CARTESIAN_POINT('Ctrl Pts',(29.2444941385794,183.002028447915,-40.5762979824596));
#12804=CARTESIAN_POINT('Ctrl Pts',(35.6711483849729,182.502028447915,-35.9444251457465));
#12805=CARTESIAN_POINT('Ctrl Pts',(40.3519323616533,182.002028447915,-29.5533069226325));
#12806=CARTESIAN_POINT('Ctrl Pts',(45.0327163383337,181.502028447915,-23.1621886995185));
#12807=CARTESIAN_POINT('Ctrl Pts',(47.5094422967239,181.002028447915,-15.6374322712211));
#12808=CARTESIAN_POINT('Ctrl Pts',(49.9861682551141,180.502028447915,-8.11267584292359));
#12809=CARTESIAN_POINT('Ctrl Pts',(50.0163970020424,180.002028447915,-0.190856796705295));
#12810=CARTESIAN_POINT('Ctrl Pts',(50.0466257489707,179.502028447915,7.730962249513));
#12811=CARTESIAN_POINT('Ctrl Pts',(47.6273982840717,179.002028447915,15.2744010708495));
#12812=CARTESIAN_POINT('Ctrl Pts',(45.2081708191727,178.502028447915,22.817839892186));
#12813=CARTESIAN_POINT('Ctrl Pts',(40.5762979824596,178.002028447915,29.2444941385794));
#12814=CARTESIAN_POINT('Ctrl Pts',(35.9444251457465,177.502028447915,35.6711483849729));
#12815=CARTESIAN_POINT('Ctrl Pts',(29.5533069226325,177.002028447915,40.3519323616533));
#12816=CARTESIAN_POINT('Ctrl Pts',(23.1621886995185,176.502028447915,45.0327163383337));
#12817=CARTESIAN_POINT('Ctrl Pts',(15.6374322712211,176.002028447915,47.5094422967239));
#12818=CARTESIAN_POINT('Ctrl Pts',(8.11267584292359,175.502028447915,49.9861682551141));
#12819=CARTESIAN_POINT('Ctrl Pts',(0.190856796705285,175.002028447915,50.0163970020424));
#12820=CARTESIAN_POINT('Ctrl Pts',(0.190856796705285,235.002028447915,50.0163970020424));
#12821=CARTESIAN_POINT('Ctrl Pts',(-7.73096224951301,234.502028447915,50.0466257489707));
#12822=CARTESIAN_POINT('Ctrl Pts',(-15.2744010708495,234.002028447915,47.6273982840717));
#12823=CARTESIAN_POINT('Ctrl Pts',(-22.817839892186,233.502028447915,45.2081708191727));
#12824=CARTESIAN_POINT('Ctrl Pts',(-29.2444941385794,233.002028447915,40.5762979824596));
#12825=CARTESIAN_POINT('Ctrl Pts',(-35.6711483849729,232.502028447915,35.9444251457465));
#12826=CARTESIAN_POINT('Ctrl Pts',(-40.3519323616533,232.002028447915,29.5533069226325));
#12827=CARTESIAN_POINT('Ctrl Pts',(-45.0327163383337,231.502028447915,23.1621886995185));
#12828=CARTESIAN_POINT('Ctrl Pts',(-47.5094422967239,231.002028447915,15.6374322712211));
#12829=CARTESIAN_POINT('Ctrl Pts',(-49.9861682551141,230.502028447915,8.11267584292358));
#12830=CARTESIAN_POINT('Ctrl Pts',(-50.0163970020424,230.002028447915,0.190856796705288));
#12831=CARTESIAN_POINT('Ctrl Pts',(-50.0466257489707,229.502028447915,-7.73096224951301));
#12832=CARTESIAN_POINT('Ctrl Pts',(-47.6273982840717,229.002028447915,-15.2744010708495));
#12833=CARTESIAN_POINT('Ctrl Pts',(-45.2081708191727,228.502028447915,-22.817839892186));
#12834=CARTESIAN_POINT('Ctrl Pts',(-40.5762979824596,228.002028447915,-29.2444941385794));
#12835=CARTESIAN_POINT('Ctrl Pts',(-35.9444251457465,227.502028447915,-35.6711483849729));
#12836=CARTESIAN_POINT('Ctrl Pts',(-29.5533069226325,227.002028447915,-40.3519323616533));
#12837=CARTESIAN_POINT('Ctrl Pts',(-23.1621886995185,226.502028447915,-45.0327163383337));
#12838=CARTESIAN_POINT('Ctrl Pts',(-15.6374322712211,226.002028447915,-47.5094422967239));
#12839=CARTESIAN_POINT('Ctrl Pts',(-8.11267584292359,225.502028447915,-49.9861682551141));
#12840=CARTESIAN_POINT('Ctrl Pts',(-0.190856796705292,225.002028447915,
-50.0163970020424));
#12841=CARTESIAN_POINT('Ctrl Pts',(7.730962249513,224.502028447915,-50.0466257489707));
#12842=CARTESIAN_POINT('Ctrl Pts',(15.2744010708495,224.002028447915,-47.6273982840717));
#12843=CARTESIAN_POINT('Ctrl Pts',(22.817839892186,223.502028447915,-45.2081708191727));
#12844=CARTESIAN_POINT('Ctrl Pts',(29.2444941385794,223.002028447915,-40.5762979824596));
#12845=CARTESIAN_POINT('Ctrl Pts',(35.6711483849729,222.502028447915,-35.9444251457465));
#12846=CARTESIAN_POINT('Ctrl Pts',(40.3519323616533,222.002028447915,-29.5533069226325));
#12847=CARTESIAN_POINT('Ctrl Pts',(45.0327163383337,221.502028447915,-23.1621886995185));
#12848=CARTESIAN_POINT('Ctrl Pts',(47.5094422967239,221.002028447915,-15.6374322712211));
#12849=CARTESIAN_POINT('Ctrl Pts',(49.9861682551141,220.502028447915,-8.11267584292359));
#12850=CARTESIAN_POINT('Ctrl Pts',(50.0163970020424,220.002028447915,-0.190856796705295));
#12851=CARTESIAN_POINT('Ctrl Pts',(50.0466257489707,219.502028447915,7.730962249513));
#12852=CARTESIAN_POINT('Ctrl Pts',(47.6273982840717,219.002028447915,15.2744010708495));
#12853=CARTESIAN_POINT('Ctrl Pts',(45.2081708191727,218.502028447915,22.817839892186));
#12854=CARTESIAN_POINT('Ctrl Pts',(40.5762979824596,218.002028447915,29.2444941385794));
#12855=CARTESIAN_POINT('Ctrl Pts',(35.9444251457465,217.502028447915,35.6711483849729));
#12856=CARTESIAN_POINT('Ctrl Pts',(29.5533069226325,217.002028447915,40.3519323616533));
#12857=CARTESIAN_POINT('Ctrl Pts',(23.1621886995185,216.502028447915,45.0327163383337));
#12858=CARTESIAN_POINT('Ctrl Pts',(15.6374322712211,216.002028447915,47.5094422967239));
#12859=CARTESIAN_POINT('Ctrl Pts',(8.11267584292359,215.502028447915,49.9861682551141));
#12860=CARTESIAN_POINT('Ctrl Pts',(0.190856796705285,215.002028447915,50.0163970020424));
#12861=CARTESIAN_POINT('Ctrl Pts',(-7.73096224951301,214.502028447915,50.0466257489707));
#12862=CARTESIAN_POINT('Ctrl Pts',(-15.2744010708495,214.002028447915,47.6273982840717));
#12863=CARTESIAN_POINT('Ctrl Pts',(-22.817839892186,213.502028447915,45.2081708191727));
#12864=CARTESIAN_POINT('Ctrl Pts',(-29.2444941385794,213.002028447915,40.5762979824596));
#12865=CARTESIAN_POINT('Ctrl Pts',(-35.6711483849729,212.502028447915,35.9444251457465));
#12866=CARTESIAN_POINT('Ctrl Pts',(-40.3519323616533,212.002028447915,29.5533069226325));
#12867=CARTESIAN_POINT('Ctrl Pts',(-45.0327163383337,211.502028447915,23.1621886995185));
#12868=CARTESIAN_POINT('Ctrl Pts',(-47.5094422967239,211.002028447915,15.6374322712211));
#12869=CARTESIAN_POINT('Ctrl Pts',(-49.9861682551141,210.502028447915,8.11267584292358));
#12870=CARTESIAN_POINT('Ctrl Pts',(-50.0163970020424,210.002028447915,0.190856796705288));
#12871=CARTESIAN_POINT('Ctrl Pts',(-50.0466257489707,209.502028447915,-7.73096224951301));
#12872=CARTESIAN_POINT('Ctrl Pts',(-47.6273982840717,209.002028447915,-15.2744010708495));
#12873=CARTESIAN_POINT('Ctrl Pts',(-45.2081708191727,208.502028447915,-22.817839892186));
#12874=CARTESIAN_POINT('Ctrl Pts',(-40.5762979824596,208.002028447915,-29.2444941385794));
#12875=CARTESIAN_POINT('Ctrl Pts',(-35.9444251457465,207.502028447915,-35.6711483849729));
#12876=CARTESIAN_POINT('Ctrl Pts',(-29.5533069226325,207.002028447915,-40.3519323616533));
#12877=CARTESIAN_POINT('Ctrl Pts',(-23.1621886995185,206.502028447915,-45.0327163383337));
#12878=CARTESIAN_POINT('Ctrl Pts',(-15.6374322712211,206.002028447915,-47.5094422967239));
#12879=CARTESIAN_POINT('Ctrl Pts',(-8.11267584292359,205.502028447915,-49.9861682551141));
#12880=CARTESIAN_POINT('Ctrl Pts',(-0.190856796705292,205.002028447915,
-50.0163970020424));
#12881=CARTESIAN_POINT('Ctrl Pts',(7.730962249513,204.502028447915,-50.0466257489707));
#12882=CARTESIAN_POINT('Ctrl Pts',(15.2744010708495,204.002028447915,-47.6273982840717));
#12883=CARTESIAN_POINT('Ctrl Pts',(22.817839892186,203.502028447915,-45.2081708191727));
#12884=CARTESIAN_POINT('Ctrl Pts',(29.2444941385794,203.002028447915,-40.5762979824596));
#12885=CARTESIAN_POINT('Ctrl Pts',(35.6711483849729,202.502028447915,-35.9444251457465));
#12886=CARTESIAN_POINT('Ctrl Pts',(40.3519323616533,202.002028447915,-29.5533069226325));
#12887=CARTESIAN_POINT('Ctrl Pts',(45.0327163383337,201.502028447915,-23.1621886995185));
#12888=CARTESIAN_POINT('Ctrl Pts',(47.5094422967239,201.002028447915,-15.6374322712211));
#12889=CARTESIAN_POINT('Ctrl Pts',(49.9861682551141,200.502028447915,-8.11267584292359));
#12890=CARTESIAN_POINT('Ctrl Pts',(50.0163970020424,200.002028447915,-0.190856796705295));
#12891=CARTESIAN_POINT('Ctrl Pts',(50.0466257489707,199.502028447915,7.730962249513));
#12892=CARTESIAN_POINT('Ctrl Pts',(47.6273982840717,199.002028447915,15.2744010708495));
#12893=CARTESIAN_POINT('Ctrl Pts',(45.2081708191727,198.502028447915,22.817839892186));
#12894=CARTESIAN_POINT('Ctrl Pts',(40.5762979824596,198.002028447915,29.2444941385794));
#12895=CARTESIAN_POINT('Ctrl Pts',(35.9444251457465,197.502028447915,35.6711483849729));
#12896=CARTESIAN_POINT('Ctrl Pts',(29.5533069226325,197.002028447915,40.3519323616533));
#12897=CARTESIAN_POINT('Ctrl Pts',(23.1621886995185,196.502028447915,45.0327163383337));
#12898=CARTESIAN_POINT('Ctrl Pts',(15.6374322712211,196.002028447915,47.5094422967239));
#12899=CARTESIAN_POINT('Ctrl Pts',(8.11267584292359,195.502028447915,49.9861682551141));
#12900=CARTESIAN_POINT('Ctrl Pts',(0.190856796705285,195.002028447915,50.0163970020424));
#12901=CARTESIAN_POINT('Ctrl Pts',(-7.73096224951301,194.502028447915,50.0466257489707));
#12902=CARTESIAN_POINT('Ctrl Pts',(-15.2744010708495,194.002028447915,47.6273982840717));
#12903=CARTESIAN_POINT('Ctrl Pts',(-22.817839892186,193.502028447915,45.2081708191727));
#12904=CARTESIAN_POINT('Ctrl Pts',(-29.2444941385794,193.002028447915,40.5762979824596));
#12905=CARTESIAN_POINT('Ctrl Pts',(-35.6711483849729,192.502028447915,35.9444251457465));
#12906=CARTESIAN_POINT('Ctrl Pts',(-40.3519323616533,192.002028447915,29.5533069226325));
#12907=CARTESIAN_POINT('Ctrl Pts',(-45.0327163383337,191.502028447915,23.1621886995185));
#12908=CARTESIAN_POINT('Ctrl Pts',(-47.5094422967239,191.002028447915,15.6374322712211));
#12909=CARTESIAN_POINT('Ctrl Pts',(-49.9861682551141,190.502028447915,8.11267584292358));
#12910=CARTESIAN_POINT('Ctrl Pts',(-50.0163970020424,190.002028447915,0.190856796705288));
#12911=CARTESIAN_POINT('Ctrl Pts',(-50.0466257489707,189.502028447915,-7.73096224951301));
#12912=CARTESIAN_POINT('Ctrl Pts',(-47.6273982840717,189.002028447915,-15.2744010708495));
#12913=CARTESIAN_POINT('Ctrl Pts',(-45.2081708191727,188.502028447915,-22.817839892186));
#12914=CARTESIAN_POINT('Ctrl Pts',(-40.5762979824596,188.002028447915,-29.2444941385794));
#12915=CARTESIAN_POINT('Ctrl Pts',(-35.9444251457465,187.502028447915,-35.6711483849729));
#12916=CARTESIAN_POINT('Ctrl Pts',(-29.5533069226325,187.002028447915,-40.3519323616533));
#12917=CARTESIAN_POINT('Ctrl Pts',(-23.1621886995185,186.502028447915,-45.0327163383337));
#12918=CARTESIAN_POINT('Ctrl Pts',(-15.6374322712211,186.002028447915,-47.5094422967239));
#12919=CARTESIAN_POINT('Ctrl Pts',(-8.11267584292359,185.502028447915,-49.9861682551141));
#12920=CARTESIAN_POINT('Ctrl Pts',(-0.190856796705292,185.002028447915,
-50.0163970020424));
#12921=CARTESIAN_POINT('Ctrl Pts',(7.730962249513,184.502028447915,-50.0466257489707));
#12922=CARTESIAN_POINT('Ctrl Pts',(15.2744010708495,184.002028447915,-47.6273982840717));
#12923=CARTESIAN_POINT('Ctrl Pts',(22.817839892186,183.502028447915,-45.2081708191727));
#12924=CARTESIAN_POINT('Ctrl Pts',(29.2444941385794,183.002028447915,-40.5762979824596));
#12925=CARTESIAN_POINT('Ctrl Pts',(35.6711483849729,182.502028447915,-35.9444251457465));
#12926=CARTESIAN_POINT('Ctrl Pts',(40.3519323616533,182.002028447915,-29.5533069226325));
#12927=CARTESIAN_POINT('Ctrl Pts',(45.0327163383337,181.502028447915,-23.1621886995185));
#12928=CARTESIAN_POINT('Ctrl Pts',(47.5094422967239,181.002028447915,-15.6374322712211));
#12929=CARTESIAN_POINT('Ctrl Pts',(49.9861682551141,180.502028447915,-8.11267584292359));
#12930=CARTESIAN_POINT('Ctrl Pts',(50.0163970020424,180.002028447915,-0.190856796705295));
#12931=CARTESIAN_POINT('Ctrl Pts',(50.0466257489707,179.502028447915,7.730962249513));
#12932=CARTESIAN_POINT('Ctrl Pts',(47.6273982840717,179.002028447915,15.2744010708495));
#12933=CARTESIAN_POINT('Ctrl Pts',(45.2081708191727,178.502028447915,22.817839892186));
#12934=CARTESIAN_POINT('Ctrl Pts',(40.5762979824596,178.002028447915,29.2444941385794));
#12935=CARTESIAN_POINT('Ctrl Pts',(35.9444251457465,177.502028447915,35.6711483849729));
#12936=CARTESIAN_POINT('Ctrl Pts',(29.5533069226325,177.002028447915,40.3519323616533));
#12937=CARTESIAN_POINT('Ctrl Pts',(23.1621886995185,176.502028447915,45.0327163383337));
#12938=CARTESIAN_POINT('Ctrl Pts',(15.6374322712211,176.002028447915,47.5094422967239));
#12939=CARTESIAN_POINT('Ctrl Pts',(8.11267584292359,175.502028447915,49.9861682551141));
#12940=CARTESIAN_POINT('Ctrl Pts',(0.190856796705285,175.002028447915,50.0163970020424));
#12941=CARTESIAN_POINT('Ctrl Pts',(0.000256710972400879,237.995967593475,
50.0163970020424));
#12942=CARTESIAN_POINT('Ctrl Pts',(-7.92156233524589,237.495967593475,50.0164376610661));
#12943=CARTESIAN_POINT('Ctrl Pts',(-15.4556725243922,236.995967593475,47.5684996184509));
#12944=CARTESIAN_POINT('Ctrl Pts',(-22.9897827135384,236.495967593475,45.1205615758357));
#12945=CARTESIAN_POINT('Ctrl Pts',(-29.3986928470667,235.995967593475,40.4642660629801));
#12946=CARTESIAN_POINT('Ctrl Pts',(-35.8076029805949,235.495967593475,35.8079705501245));
#12947=CARTESIAN_POINT('Ctrl Pts',(-40.4639642811328,234.995967593475,29.3991082141453));
#12948=CARTESIAN_POINT('Ctrl Pts',(-45.1203255816707,234.495967593475,22.990245878166));
#12949=CARTESIAN_POINT('Ctrl Pts',(-47.5683409623447,233.995967593475,15.4561608176784));
#12950=CARTESIAN_POINT('Ctrl Pts',(-50.0163563430187,233.495967593475,7.9220757571907));
#12951=CARTESIAN_POINT('Ctrl Pts',(-50.0163970020424,232.995967593475,0.000256710972403942));
#12952=CARTESIAN_POINT('Ctrl Pts',(-50.0164376610661,232.495967593475,-7.92156233524589));
#12953=CARTESIAN_POINT('Ctrl Pts',(-47.5684996184509,231.995967593475,-15.4556725243922));
#12954=CARTESIAN_POINT('Ctrl Pts',(-45.1205615758357,231.495967593475,-22.9897827135384));
#12955=CARTESIAN_POINT('Ctrl Pts',(-40.4642660629801,230.995967593475,-29.3986928470667));
#12956=CARTESIAN_POINT('Ctrl Pts',(-35.8079705501245,230.495967593475,-35.8076029805949));
#12957=CARTESIAN_POINT('Ctrl Pts',(-29.3991082141453,229.995967593475,-40.4639642811328));
#12958=CARTESIAN_POINT('Ctrl Pts',(-22.9902458781661,229.495967593475,-45.1203255816707));
#12959=CARTESIAN_POINT('Ctrl Pts',(-15.4561608176784,228.995967593475,-47.5683409623447));
#12960=CARTESIAN_POINT('Ctrl Pts',(-7.92207575719071,228.495967593475,-50.0163563430187));
#12961=CARTESIAN_POINT('Ctrl Pts',(-0.000256710972407005,227.995967593475,
-50.0163970020424));
#12962=CARTESIAN_POINT('Ctrl Pts',(7.92156233524589,227.495967593475,-50.0164376610661));
#12963=CARTESIAN_POINT('Ctrl Pts',(15.4556725243922,226.995967593475,-47.5684996184509));
#12964=CARTESIAN_POINT('Ctrl Pts',(22.9897827135384,226.495967593475,-45.1205615758357));
#12965=CARTESIAN_POINT('Ctrl Pts',(29.3986928470667,225.995967593475,-40.4642660629801));
#12966=CARTESIAN_POINT('Ctrl Pts',(35.8076029805949,225.495967593475,-35.8079705501245));
#12967=CARTESIAN_POINT('Ctrl Pts',(40.4639642811328,224.995967593475,-29.3991082141453));
#12968=CARTESIAN_POINT('Ctrl Pts',(45.1203255816707,224.495967593475,-22.9902458781661));
#12969=CARTESIAN_POINT('Ctrl Pts',(47.5683409623447,223.995967593475,-15.4561608176784));
#12970=CARTESIAN_POINT('Ctrl Pts',(50.0163563430187,223.495967593475,-7.92207575719071));
#12971=CARTESIAN_POINT('Ctrl Pts',(50.0163970020424,222.995967593475,-0.000256710972410067));
#12972=CARTESIAN_POINT('Ctrl Pts',(50.0164376610661,222.495967593475,7.92156233524589));
#12973=CARTESIAN_POINT('Ctrl Pts',(47.5684996184509,221.995967593475,15.4556725243922));
#12974=CARTESIAN_POINT('Ctrl Pts',(45.1205615758358,221.495967593475,22.9897827135384));
#12975=CARTESIAN_POINT('Ctrl Pts',(40.4642660629801,220.995967593475,29.3986928470667));
#12976=CARTESIAN_POINT('Ctrl Pts',(35.8079705501245,220.495967593475,35.8076029805949));
#12977=CARTESIAN_POINT('Ctrl Pts',(29.3991082141453,219.995967593475,40.4639642811328));
#12978=CARTESIAN_POINT('Ctrl Pts',(22.9902458781661,219.495967593475,45.1203255816707));
#12979=CARTESIAN_POINT('Ctrl Pts',(15.4561608176784,218.995967593475,47.5683409623447));
#12980=CARTESIAN_POINT('Ctrl Pts',(7.92207575719071,218.495967593475,50.0163563430187));
#12981=CARTESIAN_POINT('Ctrl Pts',(0.000256710972400879,217.995967593475,
50.0163970020424));
#12982=CARTESIAN_POINT('Ctrl Pts',(-7.92156233524589,217.495967593475,50.0164376610661));
#12983=CARTESIAN_POINT('Ctrl Pts',(-15.4556725243922,216.995967593475,47.5684996184509));
#12984=CARTESIAN_POINT('Ctrl Pts',(-22.9897827135384,216.495967593475,45.1205615758357));
#12985=CARTESIAN_POINT('Ctrl Pts',(-29.3986928470667,215.995967593475,40.4642660629801));
#12986=CARTESIAN_POINT('Ctrl Pts',(-35.8076029805949,215.495967593475,35.8079705501245));
#12987=CARTESIAN_POINT('Ctrl Pts',(-40.4639642811328,214.995967593475,29.3991082141453));
#12988=CARTESIAN_POINT('Ctrl Pts',(-45.1203255816707,214.495967593475,22.990245878166));
#12989=CARTESIAN_POINT('Ctrl Pts',(-47.5683409623447,213.995967593475,15.4561608176784));
#12990=CARTESIAN_POINT('Ctrl Pts',(-50.0163563430187,213.495967593475,7.9220757571907));
#12991=CARTESIAN_POINT('Ctrl Pts',(-50.0163970020424,212.995967593475,0.000256710972403942));
#12992=CARTESIAN_POINT('Ctrl Pts',(-50.0164376610661,212.495967593475,-7.92156233524589));
#12993=CARTESIAN_POINT('Ctrl Pts',(-47.5684996184509,211.995967593475,-15.4556725243922));
#12994=CARTESIAN_POINT('Ctrl Pts',(-45.1205615758357,211.495967593475,-22.9897827135384));
#12995=CARTESIAN_POINT('Ctrl Pts',(-40.4642660629801,210.995967593475,-29.3986928470667));
#12996=CARTESIAN_POINT('Ctrl Pts',(-35.8079705501245,210.495967593475,-35.8076029805949));
#12997=CARTESIAN_POINT('Ctrl Pts',(-29.3991082141453,209.995967593475,-40.4639642811328));
#12998=CARTESIAN_POINT('Ctrl Pts',(-22.9902458781661,209.495967593475,-45.1203255816707));
#12999=CARTESIAN_POINT('Ctrl Pts',(-15.4561608176784,208.995967593475,-47.5683409623447));
#13000=CARTESIAN_POINT('Ctrl Pts',(-7.92207575719071,208.495967593475,-50.0163563430187));
#13001=CARTESIAN_POINT('Ctrl Pts',(-0.000256710972407005,207.995967593475,
-50.0163970020424));
#13002=CARTESIAN_POINT('Ctrl Pts',(7.92156233524589,207.495967593475,-50.0164376610661));
#13003=CARTESIAN_POINT('Ctrl Pts',(15.4556725243922,206.995967593475,-47.5684996184509));
#13004=CARTESIAN_POINT('Ctrl Pts',(22.9897827135384,206.495967593475,-45.1205615758357));
#13005=CARTESIAN_POINT('Ctrl Pts',(29.3986928470667,205.995967593475,-40.4642660629801));
#13006=CARTESIAN_POINT('Ctrl Pts',(35.8076029805949,205.495967593475,-35.8079705501245));
#13007=CARTESIAN_POINT('Ctrl Pts',(40.4639642811328,204.995967593475,-29.3991082141453));
#13008=CARTESIAN_POINT('Ctrl Pts',(45.1203255816707,204.495967593475,-22.9902458781661));
#13009=CARTESIAN_POINT('Ctrl Pts',(47.5683409623447,203.995967593475,-15.4561608176784));
#13010=CARTESIAN_POINT('Ctrl Pts',(50.0163563430187,203.495967593475,-7.92207575719071));
#13011=CARTESIAN_POINT('Ctrl Pts',(50.0163970020424,202.995967593475,-0.000256710972410067));
#13012=CARTESIAN_POINT('Ctrl Pts',(50.0164376610661,202.495967593475,7.92156233524589));
#13013=CARTESIAN_POINT('Ctrl Pts',(47.5684996184509,201.995967593475,15.4556725243922));
#13014=CARTESIAN_POINT('Ctrl Pts',(45.1205615758358,201.495967593475,22.9897827135384));
#13015=CARTESIAN_POINT('Ctrl Pts',(40.4642660629801,200.995967593475,29.3986928470667));
#13016=CARTESIAN_POINT('Ctrl Pts',(35.8079705501245,200.495967593475,35.8076029805949));
#13017=CARTESIAN_POINT('Ctrl Pts',(29.3991082141453,199.995967593475,40.4639642811328));
#13018=CARTESIAN_POINT('Ctrl Pts',(22.9902458781661,199.495967593475,45.1203255816707));
#13019=CARTESIAN_POINT('Ctrl Pts',(15.4561608176784,198.995967593475,47.5683409623447));
#13020=CARTESIAN_POINT('Ctrl Pts',(7.92207575719071,198.495967593475,50.0163563430187));
#13021=CARTESIAN_POINT('Ctrl Pts',(0.000256710972400879,197.995967593475,
50.0163970020424));
#13022=CARTESIAN_POINT('Ctrl Pts',(-7.92156233524589,197.495967593475,50.0164376610661));
#13023=CARTESIAN_POINT('Ctrl Pts',(-15.4556725243922,196.995967593475,47.5684996184509));
#13024=CARTESIAN_POINT('Ctrl Pts',(-22.9897827135384,196.495967593475,45.1205615758357));
#13025=CARTESIAN_POINT('Ctrl Pts',(-29.3986928470667,195.995967593475,40.4642660629801));
#13026=CARTESIAN_POINT('Ctrl Pts',(-35.8076029805949,195.495967593475,35.8079705501245));
#13027=CARTESIAN_POINT('Ctrl Pts',(-40.4639642811328,194.995967593475,29.3991082141453));
#13028=CARTESIAN_POINT('Ctrl Pts',(-45.1203255816707,194.495967593475,22.990245878166));
#13029=CARTESIAN_POINT('Ctrl Pts',(-47.5683409623447,193.995967593475,15.4561608176784));
#13030=CARTESIAN_POINT('Ctrl Pts',(-50.0163563430187,193.495967593475,7.9220757571907));
#13031=CARTESIAN_POINT('Ctrl Pts',(-50.0163970020424,192.995967593475,0.000256710972403942));
#13032=CARTESIAN_POINT('Ctrl Pts',(-50.0164376610661,192.495967593475,-7.92156233524589));
#13033=CARTESIAN_POINT('Ctrl Pts',(-47.5684996184509,191.995967593475,-15.4556725243922));
#13034=CARTESIAN_POINT('Ctrl Pts',(-45.1205615758357,191.495967593475,-22.9897827135384));
#13035=CARTESIAN_POINT('Ctrl Pts',(-40.4642660629801,190.995967593475,-29.3986928470667));
#13036=CARTESIAN_POINT('Ctrl Pts',(-35.8079705501245,190.495967593475,-35.8076029805949));
#13037=CARTESIAN_POINT('Ctrl Pts',(-29.3991082141453,189.995967593475,-40.4639642811328));
#13038=CARTESIAN_POINT('Ctrl Pts',(-22.9902458781661,189.495967593475,-45.1203255816707));
#13039=CARTESIAN_POINT('Ctrl Pts',(-15.4561608176784,188.995967593475,-47.5683409623447));
#13040=CARTESIAN_POINT('Ctrl Pts',(-7.92207575719071,188.495967593475,-50.0163563430187));
#13041=CARTESIAN_POINT('Ctrl Pts',(-0.000256710972407005,187.995967593475,
-50.0163970020424));
#13042=CARTESIAN_POINT('Ctrl Pts',(7.92156233524589,187.495967593475,-50.0164376610661));
#13043=CARTESIAN_POINT('Ctrl Pts',(15.4556725243922,186.995967593475,-47.5684996184509));
#13044=CARTESIAN_POINT('Ctrl Pts',(22.9897827135384,186.495967593475,-45.1205615758357));
#13045=CARTESIAN_POINT('Ctrl Pts',(29.3986928470667,185.995967593475,-40.4642660629801));
#13046=CARTESIAN_POINT('Ctrl Pts',(35.8076029805949,185.495967593475,-35.8079705501245));
#13047=CARTESIAN_POINT('Ctrl Pts',(40.4639642811328,184.995967593475,-29.3991082141453));
#13048=CARTESIAN_POINT('Ctrl Pts',(45.1203255816707,184.495967593475,-22.9902458781661));
#13049=CARTESIAN_POINT('Ctrl Pts',(47.5683409623447,183.995967593475,-15.4561608176784));
#13050=CARTESIAN_POINT('Ctrl Pts',(50.0163563430187,183.495967593475,-7.92207575719071));
#13051=CARTESIAN_POINT('Ctrl Pts',(50.0163970020424,182.995967593475,-0.000256710972410067));
#13052=CARTESIAN_POINT('Ctrl Pts',(50.0164376610661,182.495967593475,7.92156233524589));
#13053=CARTESIAN_POINT('Ctrl Pts',(47.5684996184509,181.995967593475,15.4556725243922));
#13054=CARTESIAN_POINT('Ctrl Pts',(45.1205615758358,181.495967593475,22.9897827135384));
#13055=CARTESIAN_POINT('Ctrl Pts',(40.4642660629801,180.995967593475,29.3986928470667));
#13056=CARTESIAN_POINT('Ctrl Pts',(35.8079705501245,180.495967593475,35.8076029805949));
#13057=CARTESIAN_POINT('Ctrl Pts',(29.3991082141453,179.995967593475,40.4639642811328));
#13058=CARTESIAN_POINT('Ctrl Pts',(22.9902458781661,179.495967593475,45.1203255816707));
#13059=CARTESIAN_POINT('Ctrl Pts',(15.4561608176784,178.995967593475,47.5683409623447));
#13060=CARTESIAN_POINT('Ctrl Pts',(7.92207575719071,178.495967593475,50.0163563430187));
#13061=CARTESIAN_POINT('Ctrl Pts',(0.000256710972400879,177.995967593475,
50.0163970020424));
#13062=CARTESIAN_POINT('Ctrl Pts',(0.00025671097240121,237.995967593475,
7.5));
#13063=CARTESIAN_POINT('Ctrl Pts',(-1.18762659146162,237.495967593475,7.50004065902369));
#13064=CARTESIAN_POINT('Ctrl Pts',(-2.317383311169,236.995967593475,7.13300320026677));
#13065=CARTESIAN_POINT('Ctrl Pts',(-3.44714003087638,236.495967593475,6.76596574150984));
#13066=CARTESIAN_POINT('Ctrl Pts',(-4.40818170865423,235.995967593475,6.06777834873578));
#13067=CARTESIAN_POINT('Ctrl Pts',(-5.36922338643209,235.495967593475,5.36959095596173));
#13068=CARTESIAN_POINT('Ctrl Pts',(-6.06747656688843,234.995967593475,4.40859707573286));
#13069=CARTESIAN_POINT('Ctrl Pts',(-6.76572974734476,234.495967593475,3.447603195504));
#13070=CARTESIAN_POINT('Ctrl Pts',(-7.13284454416054,233.995967593475,2.31787160445521));
#13071=CARTESIAN_POINT('Ctrl Pts',(-7.49995934097631,233.495967593475,1.18814001340642));
#13072=CARTESIAN_POINT('Ctrl Pts',(-7.5,232.995967593475,0.000256710972401669));
#13073=CARTESIAN_POINT('Ctrl Pts',(-7.50004065902369,232.495967593475,-1.18762659146162));
#13074=CARTESIAN_POINT('Ctrl Pts',(-7.13300320026677,231.995967593475,-2.317383311169));
#13075=CARTESIAN_POINT('Ctrl Pts',(-6.76596574150984,231.495967593475,-3.44714003087638));
#13076=CARTESIAN_POINT('Ctrl Pts',(-6.06777834873578,230.995967593475,-4.40818170865423));
#13077=CARTESIAN_POINT('Ctrl Pts',(-5.36959095596173,230.495967593475,-5.36922338643209));
#13078=CARTESIAN_POINT('Ctrl Pts',(-4.40859707573286,229.995967593475,-6.06747656688843));
#13079=CARTESIAN_POINT('Ctrl Pts',(-3.447603195504,229.495967593475,-6.76572974734476));
#13080=CARTESIAN_POINT('Ctrl Pts',(-2.31787160445521,228.995967593475,-7.13284454416054));
#13081=CARTESIAN_POINT('Ctrl Pts',(-1.18814001340642,228.495967593475,-7.49995934097631));
#13082=CARTESIAN_POINT('Ctrl Pts',(-0.000256710972402128,227.995967593475,
-7.5));
#13083=CARTESIAN_POINT('Ctrl Pts',(1.18762659146162,227.495967593475,-7.50004065902369));
#13084=CARTESIAN_POINT('Ctrl Pts',(2.317383311169,226.995967593475,-7.13300320026677));
#13085=CARTESIAN_POINT('Ctrl Pts',(3.44714003087638,226.495967593475,-6.76596574150984));
#13086=CARTESIAN_POINT('Ctrl Pts',(4.40818170865423,225.995967593475,-6.06777834873578));
#13087=CARTESIAN_POINT('Ctrl Pts',(5.36922338643209,225.495967593475,-5.36959095596173));
#13088=CARTESIAN_POINT('Ctrl Pts',(6.06747656688843,224.995967593475,-4.40859707573286));
#13089=CARTESIAN_POINT('Ctrl Pts',(6.76572974734476,224.495967593475,-3.447603195504));
#13090=CARTESIAN_POINT('Ctrl Pts',(7.13284454416054,223.995967593475,-2.31787160445521));
#13091=CARTESIAN_POINT('Ctrl Pts',(7.49995934097631,223.495967593475,-1.18814001340642));
#13092=CARTESIAN_POINT('Ctrl Pts',(7.5,222.995967593475,-0.000256710972402588));
#13093=CARTESIAN_POINT('Ctrl Pts',(7.50004065902369,222.495967593475,1.18762659146162));
#13094=CARTESIAN_POINT('Ctrl Pts',(7.13300320026677,221.995967593475,2.317383311169));
#13095=CARTESIAN_POINT('Ctrl Pts',(6.76596574150984,221.495967593475,3.44714003087638));
#13096=CARTESIAN_POINT('Ctrl Pts',(6.06777834873579,220.995967593475,4.40818170865423));
#13097=CARTESIAN_POINT('Ctrl Pts',(5.36959095596173,220.495967593475,5.36922338643209));
#13098=CARTESIAN_POINT('Ctrl Pts',(4.40859707573286,219.995967593475,6.06747656688843));
#13099=CARTESIAN_POINT('Ctrl Pts',(3.447603195504,219.495967593475,6.76572974734476));
#13100=CARTESIAN_POINT('Ctrl Pts',(2.31787160445521,218.995967593475,7.13284454416054));
#13101=CARTESIAN_POINT('Ctrl Pts',(1.18814001340643,218.495967593475,7.49995934097631));
#13102=CARTESIAN_POINT('Ctrl Pts',(0.00025671097240121,217.995967593475,
7.5));
#13103=CARTESIAN_POINT('Ctrl Pts',(-1.18762659146162,217.495967593475,7.50004065902369));
#13104=CARTESIAN_POINT('Ctrl Pts',(-2.317383311169,216.995967593475,7.13300320026677));
#13105=CARTESIAN_POINT('Ctrl Pts',(-3.44714003087638,216.495967593475,6.76596574150984));
#13106=CARTESIAN_POINT('Ctrl Pts',(-4.40818170865423,215.995967593475,6.06777834873578));
#13107=CARTESIAN_POINT('Ctrl Pts',(-5.36922338643209,215.495967593475,5.36959095596173));
#13108=CARTESIAN_POINT('Ctrl Pts',(-6.06747656688843,214.995967593475,4.40859707573286));
#13109=CARTESIAN_POINT('Ctrl Pts',(-6.76572974734476,214.495967593475,3.447603195504));
#13110=CARTESIAN_POINT('Ctrl Pts',(-7.13284454416054,213.995967593475,2.31787160445521));
#13111=CARTESIAN_POINT('Ctrl Pts',(-7.49995934097631,213.495967593475,1.18814001340642));
#13112=CARTESIAN_POINT('Ctrl Pts',(-7.5,212.995967593475,0.000256710972401669));
#13113=CARTESIAN_POINT('Ctrl Pts',(-7.50004065902369,212.495967593475,-1.18762659146162));
#13114=CARTESIAN_POINT('Ctrl Pts',(-7.13300320026677,211.995967593475,-2.317383311169));
#13115=CARTESIAN_POINT('Ctrl Pts',(-6.76596574150984,211.495967593475,-3.44714003087638));
#13116=CARTESIAN_POINT('Ctrl Pts',(-6.06777834873578,210.995967593475,-4.40818170865423));
#13117=CARTESIAN_POINT('Ctrl Pts',(-5.36959095596173,210.495967593475,-5.36922338643209));
#13118=CARTESIAN_POINT('Ctrl Pts',(-4.40859707573286,209.995967593475,-6.06747656688843));
#13119=CARTESIAN_POINT('Ctrl Pts',(-3.447603195504,209.495967593475,-6.76572974734476));
#13120=CARTESIAN_POINT('Ctrl Pts',(-2.31787160445521,208.995967593475,-7.13284454416054));
#13121=CARTESIAN_POINT('Ctrl Pts',(-1.18814001340642,208.495967593475,-7.49995934097631));
#13122=CARTESIAN_POINT('Ctrl Pts',(-0.000256710972402128,207.995967593475,
-7.5));
#13123=CARTESIAN_POINT('Ctrl Pts',(1.18762659146162,207.495967593475,-7.50004065902369));
#13124=CARTESIAN_POINT('Ctrl Pts',(2.317383311169,206.995967593475,-7.13300320026677));
#13125=CARTESIAN_POINT('Ctrl Pts',(3.44714003087638,206.495967593475,-6.76596574150984));
#13126=CARTESIAN_POINT('Ctrl Pts',(4.40818170865423,205.995967593475,-6.06777834873578));
#13127=CARTESIAN_POINT('Ctrl Pts',(5.36922338643209,205.495967593475,-5.36959095596173));
#13128=CARTESIAN_POINT('Ctrl Pts',(6.06747656688843,204.995967593475,-4.40859707573286));
#13129=CARTESIAN_POINT('Ctrl Pts',(6.76572974734476,204.495967593475,-3.447603195504));
#13130=CARTESIAN_POINT('Ctrl Pts',(7.13284454416054,203.995967593475,-2.31787160445521));
#13131=CARTESIAN_POINT('Ctrl Pts',(7.49995934097631,203.495967593475,-1.18814001340642));
#13132=CARTESIAN_POINT('Ctrl Pts',(7.5,202.995967593475,-0.000256710972402588));
#13133=CARTESIAN_POINT('Ctrl Pts',(7.50004065902369,202.495967593475,1.18762659146162));
#13134=CARTESIAN_POINT('Ctrl Pts',(7.13300320026677,201.995967593475,2.317383311169));
#13135=CARTESIAN_POINT('Ctrl Pts',(6.76596574150984,201.495967593475,3.44714003087638));
#13136=CARTESIAN_POINT('Ctrl Pts',(6.06777834873579,200.995967593475,4.40818170865423));
#13137=CARTESIAN_POINT('Ctrl Pts',(5.36959095596173,200.495967593475,5.36922338643209));
#13138=CARTESIAN_POINT('Ctrl Pts',(4.40859707573286,199.995967593475,6.06747656688843));
#13139=CARTESIAN_POINT('Ctrl Pts',(3.447603195504,199.495967593475,6.76572974734476));
#13140=CARTESIAN_POINT('Ctrl Pts',(2.31787160445521,198.995967593475,7.13284454416054));
#13141=CARTESIAN_POINT('Ctrl Pts',(1.18814001340643,198.495967593475,7.49995934097631));
#13142=CARTESIAN_POINT('Ctrl Pts',(0.00025671097240121,197.995967593475,
7.5));
#13143=CARTESIAN_POINT('Ctrl Pts',(-1.18762659146162,197.495967593475,7.50004065902369));
#13144=CARTESIAN_POINT('Ctrl Pts',(-2.317383311169,196.995967593475,7.13300320026677));
#13145=CARTESIAN_POINT('Ctrl Pts',(-3.44714003087638,196.495967593475,6.76596574150984));
#13146=CARTESIAN_POINT('Ctrl Pts',(-4.40818170865423,195.995967593475,6.06777834873578));
#13147=CARTESIAN_POINT('Ctrl Pts',(-5.36922338643209,195.495967593475,5.36959095596173));
#13148=CARTESIAN_POINT('Ctrl Pts',(-6.06747656688843,194.995967593475,4.40859707573286));
#13149=CARTESIAN_POINT('Ctrl Pts',(-6.76572974734476,194.495967593475,3.447603195504));
#13150=CARTESIAN_POINT('Ctrl Pts',(-7.13284454416054,193.995967593475,2.31787160445521));
#13151=CARTESIAN_POINT('Ctrl Pts',(-7.49995934097631,193.495967593475,1.18814001340642));
#13152=CARTESIAN_POINT('Ctrl Pts',(-7.5,192.995967593475,0.000256710972401669));
#13153=CARTESIAN_POINT('Ctrl Pts',(-7.50004065902369,192.495967593475,-1.18762659146162));
#13154=CARTESIAN_POINT('Ctrl Pts',(-7.13300320026677,191.995967593475,-2.317383311169));
#13155=CARTESIAN_POINT('Ctrl Pts',(-6.76596574150984,191.495967593475,-3.44714003087638));
#13156=CARTESIAN_POINT('Ctrl Pts',(-6.06777834873578,190.995967593475,-4.40818170865423));
#13157=CARTESIAN_POINT('Ctrl Pts',(-5.36959095596173,190.495967593475,-5.36922338643209));
#13158=CARTESIAN_POINT('Ctrl Pts',(-4.40859707573286,189.995967593475,-6.06747656688843));
#13159=CARTESIAN_POINT('Ctrl Pts',(-3.447603195504,189.495967593475,-6.76572974734476));
#13160=CARTESIAN_POINT('Ctrl Pts',(-2.31787160445521,188.995967593475,-7.13284454416054));
#13161=CARTESIAN_POINT('Ctrl Pts',(-1.18814001340642,188.495967593475,-7.49995934097631));
#13162=CARTESIAN_POINT('Ctrl Pts',(-0.000256710972402128,187.995967593475,
-7.5));
#13163=CARTESIAN_POINT('Ctrl Pts',(1.18762659146162,187.495967593475,-7.50004065902369));
#13164=CARTESIAN_POINT('Ctrl Pts',(2.317383311169,186.995967593475,-7.13300320026677));
#13165=CARTESIAN_POINT('Ctrl Pts',(3.44714003087638,186.495967593475,-6.76596574150984));
#13166=CARTESIAN_POINT('Ctrl Pts',(4.40818170865423,185.995967593475,-6.06777834873578));
#13167=CARTESIAN_POINT('Ctrl Pts',(5.36922338643209,185.495967593475,-5.36959095596173));
#13168=CARTESIAN_POINT('Ctrl Pts',(6.06747656688843,184.995967593475,-4.40859707573286));
#13169=CARTESIAN_POINT('Ctrl Pts',(6.76572974734476,184.495967593475,-3.447603195504));
#13170=CARTESIAN_POINT('Ctrl Pts',(7.13284454416054,183.995967593475,-2.31787160445521));
#13171=CARTESIAN_POINT('Ctrl Pts',(7.49995934097631,183.495967593475,-1.18814001340642));
#13172=CARTESIAN_POINT('Ctrl Pts',(7.5,182.995967593475,-0.000256710972402588));
#13173=CARTESIAN_POINT('Ctrl Pts',(7.50004065902369,182.495967593475,1.18762659146162));
#13174=CARTESIAN_POINT('Ctrl Pts',(7.13300320026677,181.995967593475,2.317383311169));
#13175=CARTESIAN_POINT('Ctrl Pts',(6.76596574150984,181.495967593475,3.44714003087638));
#13176=CARTESIAN_POINT('Ctrl Pts',(6.06777834873579,180.995967593475,4.40818170865423));
#13177=CARTESIAN_POINT('Ctrl Pts',(5.36959095596173,180.495967593475,5.36922338643209));
#13178=CARTESIAN_POINT('Ctrl Pts',(4.40859707573286,179.995967593475,6.06747656688843));
#13179=CARTESIAN_POINT('Ctrl Pts',(3.447603195504,179.495967593475,6.76572974734476));
#13180=CARTESIAN_POINT('Ctrl Pts',(2.31787160445521,178.995967593475,7.13284454416054));
#13181=CARTESIAN_POINT('Ctrl Pts',(1.18814001340643,178.495967593475,7.49995934097631));
#13182=CARTESIAN_POINT('Ctrl Pts',(0.00025671097240121,177.995967593475,
7.5));
#13183=CARTESIAN_POINT('Ctrl Pts',(0.000256710972400845,237.995967593475,
50.0163970020424));
#13184=CARTESIAN_POINT('Ctrl Pts',(-7.92156233524589,237.495967593475,50.0164376610661));
#13185=CARTESIAN_POINT('Ctrl Pts',(-15.4556725243922,236.995967593475,47.5684996184509));
#13186=CARTESIAN_POINT('Ctrl Pts',(-22.9897827135384,236.495967593475,45.1205615758357));
#13187=CARTESIAN_POINT('Ctrl Pts',(-29.3986928470667,235.995967593475,40.4642660629801));
#13188=CARTESIAN_POINT('Ctrl Pts',(-35.8076029805949,235.495967593475,35.8079705501245));
#13189=CARTESIAN_POINT('Ctrl Pts',(-40.4639642811328,234.995967593475,29.3991082141453));
#13190=CARTESIAN_POINT('Ctrl Pts',(-45.1203255816707,234.495967593475,22.990245878166));
#13191=CARTESIAN_POINT('Ctrl Pts',(-47.5683409623447,233.995967593475,15.4561608176784));
#13192=CARTESIAN_POINT('Ctrl Pts',(-50.0163563430187,233.495967593475,7.9220757571907));
#13193=CARTESIAN_POINT('Ctrl Pts',(-50.0163970020424,232.995967593475,0.000256710972403907));
#13194=CARTESIAN_POINT('Ctrl Pts',(-50.0164376610661,232.495967593475,-7.92156233524589));
#13195=CARTESIAN_POINT('Ctrl Pts',(-47.5684996184509,231.995967593475,-15.4556725243922));
#13196=CARTESIAN_POINT('Ctrl Pts',(-45.1205615758357,231.495967593475,-22.9897827135384));
#13197=CARTESIAN_POINT('Ctrl Pts',(-40.4642660629801,230.995967593475,-29.3986928470667));
#13198=CARTESIAN_POINT('Ctrl Pts',(-35.8079705501245,230.495967593475,-35.8076029805949));
#13199=CARTESIAN_POINT('Ctrl Pts',(-29.3991082141453,229.995967593475,-40.4639642811328));
#13200=CARTESIAN_POINT('Ctrl Pts',(-22.9902458781661,229.495967593475,-45.1203255816707));
#13201=CARTESIAN_POINT('Ctrl Pts',(-15.4561608176784,228.995967593475,-47.5683409623447));
#13202=CARTESIAN_POINT('Ctrl Pts',(-7.92207575719071,228.495967593475,-50.0163563430187));
#13203=CARTESIAN_POINT('Ctrl Pts',(-0.00025671097240697,227.995967593475,
-50.0163970020424));
#13204=CARTESIAN_POINT('Ctrl Pts',(7.92156233524589,227.495967593475,-50.0164376610661));
#13205=CARTESIAN_POINT('Ctrl Pts',(15.4556725243922,226.995967593475,-47.5684996184509));
#13206=CARTESIAN_POINT('Ctrl Pts',(22.9897827135384,226.495967593475,-45.1205615758357));
#13207=CARTESIAN_POINT('Ctrl Pts',(29.3986928470667,225.995967593475,-40.4642660629801));
#13208=CARTESIAN_POINT('Ctrl Pts',(35.8076029805949,225.495967593475,-35.8079705501245));
#13209=CARTESIAN_POINT('Ctrl Pts',(40.4639642811328,224.995967593475,-29.3991082141453));
#13210=CARTESIAN_POINT('Ctrl Pts',(45.1203255816707,224.495967593475,-22.9902458781661));
#13211=CARTESIAN_POINT('Ctrl Pts',(47.5683409623447,223.995967593475,-15.4561608176784));
#13212=CARTESIAN_POINT('Ctrl Pts',(50.0163563430187,223.495967593475,-7.92207575719071));
#13213=CARTESIAN_POINT('Ctrl Pts',(50.0163970020424,222.995967593475,-0.000256710972410033));
#13214=CARTESIAN_POINT('Ctrl Pts',(50.0164376610661,222.495967593475,7.92156233524589));
#13215=CARTESIAN_POINT('Ctrl Pts',(47.5684996184509,221.995967593475,15.4556725243922));
#13216=CARTESIAN_POINT('Ctrl Pts',(45.1205615758358,221.495967593475,22.9897827135384));
#13217=CARTESIAN_POINT('Ctrl Pts',(40.4642660629801,220.995967593475,29.3986928470667));
#13218=CARTESIAN_POINT('Ctrl Pts',(35.8079705501245,220.495967593475,35.8076029805949));
#13219=CARTESIAN_POINT('Ctrl Pts',(29.3991082141453,219.995967593475,40.4639642811328));
#13220=CARTESIAN_POINT('Ctrl Pts',(22.9902458781661,219.495967593475,45.1203255816707));
#13221=CARTESIAN_POINT('Ctrl Pts',(15.4561608176784,218.995967593475,47.5683409623447));
#13222=CARTESIAN_POINT('Ctrl Pts',(7.92207575719071,218.495967593475,50.0163563430187));
#13223=CARTESIAN_POINT('Ctrl Pts',(0.000256710972400845,217.995967593475,
50.0163970020424));
#13224=CARTESIAN_POINT('Ctrl Pts',(-7.92156233524589,217.495967593475,50.0164376610661));
#13225=CARTESIAN_POINT('Ctrl Pts',(-15.4556725243922,216.995967593475,47.5684996184509));
#13226=CARTESIAN_POINT('Ctrl Pts',(-22.9897827135384,216.495967593475,45.1205615758357));
#13227=CARTESIAN_POINT('Ctrl Pts',(-29.3986928470667,215.995967593475,40.4642660629801));
#13228=CARTESIAN_POINT('Ctrl Pts',(-35.8076029805949,215.495967593475,35.8079705501245));
#13229=CARTESIAN_POINT('Ctrl Pts',(-40.4639642811328,214.995967593475,29.3991082141453));
#13230=CARTESIAN_POINT('Ctrl Pts',(-45.1203255816707,214.495967593475,22.990245878166));
#13231=CARTESIAN_POINT('Ctrl Pts',(-47.5683409623447,213.995967593475,15.4561608176784));
#13232=CARTESIAN_POINT('Ctrl Pts',(-50.0163563430187,213.495967593475,7.9220757571907));
#13233=CARTESIAN_POINT('Ctrl Pts',(-50.0163970020424,212.995967593475,0.000256710972403907));
#13234=CARTESIAN_POINT('Ctrl Pts',(-50.0164376610661,212.495967593475,-7.92156233524589));
#13235=CARTESIAN_POINT('Ctrl Pts',(-47.5684996184509,211.995967593475,-15.4556725243922));
#13236=CARTESIAN_POINT('Ctrl Pts',(-45.1205615758357,211.495967593475,-22.9897827135384));
#13237=CARTESIAN_POINT('Ctrl Pts',(-40.4642660629801,210.995967593475,-29.3986928470667));
#13238=CARTESIAN_POINT('Ctrl Pts',(-35.8079705501245,210.495967593475,-35.8076029805949));
#13239=CARTESIAN_POINT('Ctrl Pts',(-29.3991082141453,209.995967593475,-40.4639642811328));
#13240=CARTESIAN_POINT('Ctrl Pts',(-22.9902458781661,209.495967593475,-45.1203255816707));
#13241=CARTESIAN_POINT('Ctrl Pts',(-15.4561608176784,208.995967593475,-47.5683409623447));
#13242=CARTESIAN_POINT('Ctrl Pts',(-7.92207575719071,208.495967593475,-50.0163563430187));
#13243=CARTESIAN_POINT('Ctrl Pts',(-0.00025671097240697,207.995967593475,
-50.0163970020424));
#13244=CARTESIAN_POINT('Ctrl Pts',(7.92156233524589,207.495967593475,-50.0164376610661));
#13245=CARTESIAN_POINT('Ctrl Pts',(15.4556725243922,206.995967593475,-47.5684996184509));
#13246=CARTESIAN_POINT('Ctrl Pts',(22.9897827135384,206.495967593475,-45.1205615758357));
#13247=CARTESIAN_POINT('Ctrl Pts',(29.3986928470667,205.995967593475,-40.4642660629801));
#13248=CARTESIAN_POINT('Ctrl Pts',(35.8076029805949,205.495967593475,-35.8079705501245));
#13249=CARTESIAN_POINT('Ctrl Pts',(40.4639642811328,204.995967593475,-29.3991082141453));
#13250=CARTESIAN_POINT('Ctrl Pts',(45.1203255816707,204.495967593475,-22.9902458781661));
#13251=CARTESIAN_POINT('Ctrl Pts',(47.5683409623447,203.995967593475,-15.4561608176784));
#13252=CARTESIAN_POINT('Ctrl Pts',(50.0163563430187,203.495967593475,-7.92207575719071));
#13253=CARTESIAN_POINT('Ctrl Pts',(50.0163970020424,202.995967593475,-0.000256710972410033));
#13254=CARTESIAN_POINT('Ctrl Pts',(50.0164376610661,202.495967593475,7.92156233524589));
#13255=CARTESIAN_POINT('Ctrl Pts',(47.5684996184509,201.995967593475,15.4556725243922));
#13256=CARTESIAN_POINT('Ctrl Pts',(45.1205615758358,201.495967593475,22.9897827135384));
#13257=CARTESIAN_POINT('Ctrl Pts',(40.4642660629801,200.995967593475,29.3986928470667));
#13258=CARTESIAN_POINT('Ctrl Pts',(35.8079705501245,200.495967593475,35.8076029805949));
#13259=CARTESIAN_POINT('Ctrl Pts',(29.3991082141453,199.995967593475,40.4639642811328));
#13260=CARTESIAN_POINT('Ctrl Pts',(22.9902458781661,199.495967593475,45.1203255816707));
#13261=CARTESIAN_POINT('Ctrl Pts',(15.4561608176784,198.995967593475,47.5683409623447));
#13262=CARTESIAN_POINT('Ctrl Pts',(7.92207575719071,198.495967593475,50.0163563430187));
#13263=CARTESIAN_POINT('Ctrl Pts',(0.000256710972400845,197.995967593475,
50.0163970020424));
#13264=CARTESIAN_POINT('Ctrl Pts',(-7.92156233524589,197.495967593475,50.0164376610661));
#13265=CARTESIAN_POINT('Ctrl Pts',(-15.4556725243922,196.995967593475,47.5684996184509));
#13266=CARTESIAN_POINT('Ctrl Pts',(-22.9897827135384,196.495967593475,45.1205615758357));
#13267=CARTESIAN_POINT('Ctrl Pts',(-29.3986928470667,195.995967593475,40.4642660629801));
#13268=CARTESIAN_POINT('Ctrl Pts',(-35.8076029805949,195.495967593475,35.8079705501245));
#13269=CARTESIAN_POINT('Ctrl Pts',(-40.4639642811328,194.995967593475,29.3991082141453));
#13270=CARTESIAN_POINT('Ctrl Pts',(-45.1203255816707,194.495967593475,22.990245878166));
#13271=CARTESIAN_POINT('Ctrl Pts',(-47.5683409623447,193.995967593475,15.4561608176784));
#13272=CARTESIAN_POINT('Ctrl Pts',(-50.0163563430187,193.495967593475,7.9220757571907));
#13273=CARTESIAN_POINT('Ctrl Pts',(-50.0163970020424,192.995967593475,0.000256710972403907));
#13274=CARTESIAN_POINT('Ctrl Pts',(-50.0164376610661,192.495967593475,-7.92156233524589));
#13275=CARTESIAN_POINT('Ctrl Pts',(-47.5684996184509,191.995967593475,-15.4556725243922));
#13276=CARTESIAN_POINT('Ctrl Pts',(-45.1205615758357,191.495967593475,-22.9897827135384));
#13277=CARTESIAN_POINT('Ctrl Pts',(-40.4642660629801,190.995967593475,-29.3986928470667));
#13278=CARTESIAN_POINT('Ctrl Pts',(-35.8079705501245,190.495967593475,-35.8076029805949));
#13279=CARTESIAN_POINT('Ctrl Pts',(-29.3991082141453,189.995967593475,-40.4639642811328));
#13280=CARTESIAN_POINT('Ctrl Pts',(-22.9902458781661,189.495967593475,-45.1203255816707));
#13281=CARTESIAN_POINT('Ctrl Pts',(-15.4561608176784,188.995967593475,-47.5683409623447));
#13282=CARTESIAN_POINT('Ctrl Pts',(-7.92207575719071,188.495967593475,-50.0163563430187));
#13283=CARTESIAN_POINT('Ctrl Pts',(-0.00025671097240697,187.995967593475,
-50.0163970020424));
#13284=CARTESIAN_POINT('Ctrl Pts',(7.92156233524589,187.495967593475,-50.0164376610661));
#13285=CARTESIAN_POINT('Ctrl Pts',(15.4556725243922,186.995967593475,-47.5684996184509));
#13286=CARTESIAN_POINT('Ctrl Pts',(22.9897827135384,186.495967593475,-45.1205615758357));
#13287=CARTESIAN_POINT('Ctrl Pts',(29.3986928470667,185.995967593475,-40.4642660629801));
#13288=CARTESIAN_POINT('Ctrl Pts',(35.8076029805949,185.495967593475,-35.8079705501245));
#13289=CARTESIAN_POINT('Ctrl Pts',(40.4639642811328,184.995967593475,-29.3991082141453));
#13290=CARTESIAN_POINT('Ctrl Pts',(45.1203255816707,184.495967593475,-22.9902458781661));
#13291=CARTESIAN_POINT('Ctrl Pts',(47.5683409623447,183.995967593475,-15.4561608176784));
#13292=CARTESIAN_POINT('Ctrl Pts',(50.0163563430187,183.495967593475,-7.92207575719071));
#13293=CARTESIAN_POINT('Ctrl Pts',(50.0163970020424,182.995967593475,-0.000256710972410033));
#13294=CARTESIAN_POINT('Ctrl Pts',(50.0164376610661,182.495967593475,7.92156233524589));
#13295=CARTESIAN_POINT('Ctrl Pts',(47.5684996184509,181.995967593475,15.4556725243922));
#13296=CARTESIAN_POINT('Ctrl Pts',(45.1205615758358,181.495967593475,22.9897827135384));
#13297=CARTESIAN_POINT('Ctrl Pts',(40.4642660629801,180.995967593475,29.3986928470667));
#13298=CARTESIAN_POINT('Ctrl Pts',(35.8079705501245,180.495967593475,35.8076029805949));
#13299=CARTESIAN_POINT('Ctrl Pts',(29.3991082141453,179.995967593475,40.4639642811328));
#13300=CARTESIAN_POINT('Ctrl Pts',(22.9902458781661,179.495967593475,45.1203255816707));
#13301=CARTESIAN_POINT('Ctrl Pts',(15.4561608176784,178.995967593475,47.5683409623447));
#13302=CARTESIAN_POINT('Ctrl Pts',(7.92207575719071,178.495967593475,50.0163563430187));
#13303=CARTESIAN_POINT('Ctrl Pts',(0.000256710972400845,177.995967593475,
50.0163970020424));
#13304=CARTESIAN_POINT('Ctrl Pts',(0.190856796705285,235.002028447915,50.0163970020424));
#13305=CARTESIAN_POINT('Ctrl Pts',(-7.73096224951301,234.502028447915,50.0466257489707));
#13306=CARTESIAN_POINT('Ctrl Pts',(-15.2744010708495,234.002028447915,47.6273982840717));
#13307=CARTESIAN_POINT('Ctrl Pts',(-22.817839892186,233.502028447915,45.2081708191727));
#13308=CARTESIAN_POINT('Ctrl Pts',(-29.2444941385794,233.002028447915,40.5762979824596));
#13309=CARTESIAN_POINT('Ctrl Pts',(-35.6711483849729,232.502028447915,35.9444251457465));
#13310=CARTESIAN_POINT('Ctrl Pts',(-40.3519323616533,232.002028447915,29.5533069226325));
#13311=CARTESIAN_POINT('Ctrl Pts',(-45.0327163383337,231.502028447915,23.1621886995185));
#13312=CARTESIAN_POINT('Ctrl Pts',(-47.5094422967239,231.002028447915,15.6374322712211));
#13313=CARTESIAN_POINT('Ctrl Pts',(-49.9861682551141,230.502028447915,8.11267584292358));
#13314=CARTESIAN_POINT('Ctrl Pts',(-50.0163970020424,230.002028447915,0.190856796705288));
#13315=CARTESIAN_POINT('Ctrl Pts',(-50.0466257489707,229.502028447915,-7.73096224951301));
#13316=CARTESIAN_POINT('Ctrl Pts',(-47.6273982840717,229.002028447915,-15.2744010708495));
#13317=CARTESIAN_POINT('Ctrl Pts',(-45.2081708191727,228.502028447915,-22.817839892186));
#13318=CARTESIAN_POINT('Ctrl Pts',(-40.5762979824596,228.002028447915,-29.2444941385794));
#13319=CARTESIAN_POINT('Ctrl Pts',(-35.9444251457465,227.502028447915,-35.6711483849729));
#13320=CARTESIAN_POINT('Ctrl Pts',(-29.5533069226325,227.002028447915,-40.3519323616533));
#13321=CARTESIAN_POINT('Ctrl Pts',(-23.1621886995185,226.502028447915,-45.0327163383337));
#13322=CARTESIAN_POINT('Ctrl Pts',(-15.6374322712211,226.002028447915,-47.5094422967239));
#13323=CARTESIAN_POINT('Ctrl Pts',(-8.11267584292359,225.502028447915,-49.9861682551141));
#13324=CARTESIAN_POINT('Ctrl Pts',(-0.190856796705292,225.002028447915,
-50.0163970020424));
#13325=CARTESIAN_POINT('Ctrl Pts',(7.730962249513,224.502028447915,-50.0466257489707));
#13326=CARTESIAN_POINT('Ctrl Pts',(15.2744010708495,224.002028447915,-47.6273982840717));
#13327=CARTESIAN_POINT('Ctrl Pts',(22.817839892186,223.502028447915,-45.2081708191727));
#13328=CARTESIAN_POINT('Ctrl Pts',(29.2444941385794,223.002028447915,-40.5762979824596));
#13329=CARTESIAN_POINT('Ctrl Pts',(35.6711483849729,222.502028447915,-35.9444251457465));
#13330=CARTESIAN_POINT('Ctrl Pts',(40.3519323616533,222.002028447915,-29.5533069226325));
#13331=CARTESIAN_POINT('Ctrl Pts',(45.0327163383337,221.502028447915,-23.1621886995185));
#13332=CARTESIAN_POINT('Ctrl Pts',(47.5094422967239,221.002028447915,-15.6374322712211));
#13333=CARTESIAN_POINT('Ctrl Pts',(49.9861682551141,220.502028447915,-8.11267584292359));
#13334=CARTESIAN_POINT('Ctrl Pts',(50.0163970020424,220.002028447915,-0.190856796705295));
#13335=CARTESIAN_POINT('Ctrl Pts',(50.0466257489707,219.502028447915,7.730962249513));
#13336=CARTESIAN_POINT('Ctrl Pts',(47.6273982840717,219.002028447915,15.2744010708495));
#13337=CARTESIAN_POINT('Ctrl Pts',(45.2081708191727,218.502028447915,22.817839892186));
#13338=CARTESIAN_POINT('Ctrl Pts',(40.5762979824596,218.002028447915,29.2444941385794));
#13339=CARTESIAN_POINT('Ctrl Pts',(35.9444251457465,217.502028447915,35.6711483849729));
#13340=CARTESIAN_POINT('Ctrl Pts',(29.5533069226325,217.002028447915,40.3519323616533));
#13341=CARTESIAN_POINT('Ctrl Pts',(23.1621886995185,216.502028447915,45.0327163383337));
#13342=CARTESIAN_POINT('Ctrl Pts',(15.6374322712211,216.002028447915,47.5094422967239));
#13343=CARTESIAN_POINT('Ctrl Pts',(8.11267584292359,215.502028447915,49.9861682551141));
#13344=CARTESIAN_POINT('Ctrl Pts',(0.190856796705285,215.002028447915,50.0163970020424));
#13345=CARTESIAN_POINT('Ctrl Pts',(-7.73096224951301,214.502028447915,50.0466257489707));
#13346=CARTESIAN_POINT('Ctrl Pts',(-15.2744010708495,214.002028447915,47.6273982840717));
#13347=CARTESIAN_POINT('Ctrl Pts',(-22.817839892186,213.502028447915,45.2081708191727));
#13348=CARTESIAN_POINT('Ctrl Pts',(-29.2444941385794,213.002028447915,40.5762979824596));
#13349=CARTESIAN_POINT('Ctrl Pts',(-35.6711483849729,212.502028447915,35.9444251457465));
#13350=CARTESIAN_POINT('Ctrl Pts',(-40.3519323616533,212.002028447915,29.5533069226325));
#13351=CARTESIAN_POINT('Ctrl Pts',(-45.0327163383337,211.502028447915,23.1621886995185));
#13352=CARTESIAN_POINT('Ctrl Pts',(-47.5094422967239,211.002028447915,15.6374322712211));
#13353=CARTESIAN_POINT('Ctrl Pts',(-49.9861682551141,210.502028447915,8.11267584292358));
#13354=CARTESIAN_POINT('Ctrl Pts',(-50.0163970020424,210.002028447915,0.190856796705288));
#13355=CARTESIAN_POINT('Ctrl Pts',(-50.0466257489707,209.502028447915,-7.73096224951301));
#13356=CARTESIAN_POINT('Ctrl Pts',(-47.6273982840717,209.002028447915,-15.2744010708495));
#13357=CARTESIAN_POINT('Ctrl Pts',(-45.2081708191727,208.502028447915,-22.817839892186));
#13358=CARTESIAN_POINT('Ctrl Pts',(-40.5762979824596,208.002028447915,-29.2444941385794));
#13359=CARTESIAN_POINT('Ctrl Pts',(-35.9444251457465,207.502028447915,-35.6711483849729));
#13360=CARTESIAN_POINT('Ctrl Pts',(-29.5533069226325,207.002028447915,-40.3519323616533));
#13361=CARTESIAN_POINT('Ctrl Pts',(-23.1621886995185,206.502028447915,-45.0327163383337));
#13362=CARTESIAN_POINT('Ctrl Pts',(-15.6374322712211,206.002028447915,-47.5094422967239));
#13363=CARTESIAN_POINT('Ctrl Pts',(-8.11267584292359,205.502028447915,-49.9861682551141));
#13364=CARTESIAN_POINT('Ctrl Pts',(-0.190856796705292,205.002028447915,
-50.0163970020424));
#13365=CARTESIAN_POINT('Ctrl Pts',(7.730962249513,204.502028447915,-50.0466257489707));
#13366=CARTESIAN_POINT('Ctrl Pts',(15.2744010708495,204.002028447915,-47.6273982840717));
#13367=CARTESIAN_POINT('Ctrl Pts',(22.817839892186,203.502028447915,-45.2081708191727));
#13368=CARTESIAN_POINT('Ctrl Pts',(29.2444941385794,203.002028447915,-40.5762979824596));
#13369=CARTESIAN_POINT('Ctrl Pts',(35.6711483849729,202.502028447915,-35.9444251457465));
#13370=CARTESIAN_POINT('Ctrl Pts',(40.3519323616533,202.002028447915,-29.5533069226325));
#13371=CARTESIAN_POINT('Ctrl Pts',(45.0327163383337,201.502028447915,-23.1621886995185));
#13372=CARTESIAN_POINT('Ctrl Pts',(47.5094422967239,201.002028447915,-15.6374322712211));
#13373=CARTESIAN_POINT('Ctrl Pts',(49.9861682551141,200.502028447915,-8.11267584292359));
#13374=CARTESIAN_POINT('Ctrl Pts',(50.0163970020424,200.002028447915,-0.190856796705295));
#13375=CARTESIAN_POINT('Ctrl Pts',(50.0466257489707,199.502028447915,7.730962249513));
#13376=CARTESIAN_POINT('Ctrl Pts',(47.6273982840717,199.002028447915,15.2744010708495));
#13377=CARTESIAN_POINT('Ctrl Pts',(45.2081708191727,198.502028447915,22.817839892186));
#13378=CARTESIAN_POINT('Ctrl Pts',(40.5762979824596,198.002028447915,29.2444941385794));
#13379=CARTESIAN_POINT('Ctrl Pts',(35.9444251457465,197.502028447915,35.6711483849729));
#13380=CARTESIAN_POINT('Ctrl Pts',(29.5533069226325,197.002028447915,40.3519323616533));
#13381=CARTESIAN_POINT('Ctrl Pts',(23.1621886995185,196.502028447915,45.0327163383337));
#13382=CARTESIAN_POINT('Ctrl Pts',(15.6374322712211,196.002028447915,47.5094422967239));
#13383=CARTESIAN_POINT('Ctrl Pts',(8.11267584292359,195.502028447915,49.9861682551141));
#13384=CARTESIAN_POINT('Ctrl Pts',(0.190856796705285,195.002028447915,50.0163970020424));
#13385=CARTESIAN_POINT('Ctrl Pts',(-7.73096224951301,194.502028447915,50.0466257489707));
#13386=CARTESIAN_POINT('Ctrl Pts',(-15.2744010708495,194.002028447915,47.6273982840717));
#13387=CARTESIAN_POINT('Ctrl Pts',(-22.817839892186,193.502028447915,45.2081708191727));
#13388=CARTESIAN_POINT('Ctrl Pts',(-29.2444941385794,193.002028447915,40.5762979824596));
#13389=CARTESIAN_POINT('Ctrl Pts',(-35.6711483849729,192.502028447915,35.9444251457465));
#13390=CARTESIAN_POINT('Ctrl Pts',(-40.3519323616533,192.002028447915,29.5533069226325));
#13391=CARTESIAN_POINT('Ctrl Pts',(-45.0327163383337,191.502028447915,23.1621886995185));
#13392=CARTESIAN_POINT('Ctrl Pts',(-47.5094422967239,191.002028447915,15.6374322712211));
#13393=CARTESIAN_POINT('Ctrl Pts',(-49.9861682551141,190.502028447915,8.11267584292358));
#13394=CARTESIAN_POINT('Ctrl Pts',(-50.0163970020424,190.002028447915,0.190856796705288));
#13395=CARTESIAN_POINT('Ctrl Pts',(-50.0466257489707,189.502028447915,-7.73096224951301));
#13396=CARTESIAN_POINT('Ctrl Pts',(-47.6273982840717,189.002028447915,-15.2744010708495));
#13397=CARTESIAN_POINT('Ctrl Pts',(-45.2081708191727,188.502028447915,-22.817839892186));
#13398=CARTESIAN_POINT('Ctrl Pts',(-40.5762979824596,188.002028447915,-29.2444941385794));
#13399=CARTESIAN_POINT('Ctrl Pts',(-35.9444251457465,187.502028447915,-35.6711483849729));
#13400=CARTESIAN_POINT('Ctrl Pts',(-29.5533069226325,187.002028447915,-40.3519323616533));
#13401=CARTESIAN_POINT('Ctrl Pts',(-23.1621886995185,186.502028447915,-45.0327163383337));
#13402=CARTESIAN_POINT('Ctrl Pts',(-15.6374322712211,186.002028447915,-47.5094422967239));
#13403=CARTESIAN_POINT('Ctrl Pts',(-8.11267584292359,185.502028447915,-49.9861682551141));
#13404=CARTESIAN_POINT('Ctrl Pts',(-0.190856796705292,185.002028447915,
-50.0163970020424));
#13405=CARTESIAN_POINT('Ctrl Pts',(7.730962249513,184.502028447915,-50.0466257489707));
#13406=CARTESIAN_POINT('Ctrl Pts',(15.2744010708495,184.002028447915,-47.6273982840717));
#13407=CARTESIAN_POINT('Ctrl Pts',(22.817839892186,183.502028447915,-45.2081708191727));
#13408=CARTESIAN_POINT('Ctrl Pts',(29.2444941385794,183.002028447915,-40.5762979824596));
#13409=CARTESIAN_POINT('Ctrl Pts',(35.6711483849729,182.502028447915,-35.9444251457465));
#13410=CARTESIAN_POINT('Ctrl Pts',(40.3519323616533,182.002028447915,-29.5533069226325));
#13411=CARTESIAN_POINT('Ctrl Pts',(45.0327163383337,181.502028447915,-23.1621886995185));
#13412=CARTESIAN_POINT('Ctrl Pts',(47.5094422967239,181.002028447915,-15.6374322712211));
#13413=CARTESIAN_POINT('Ctrl Pts',(49.9861682551141,180.502028447915,-8.11267584292359));
#13414=CARTESIAN_POINT('Ctrl Pts',(50.0163970020424,180.002028447915,-0.190856796705295));
#13415=CARTESIAN_POINT('Ctrl Pts',(50.0466257489707,179.502028447915,7.730962249513));
#13416=CARTESIAN_POINT('Ctrl Pts',(47.6273982840717,179.002028447915,15.2744010708495));
#13417=CARTESIAN_POINT('Ctrl Pts',(45.2081708191727,178.502028447915,22.817839892186));
#13418=CARTESIAN_POINT('Ctrl Pts',(40.5762979824596,178.002028447915,29.2444941385794));
#13419=CARTESIAN_POINT('Ctrl Pts',(35.9444251457465,177.502028447915,35.6711483849729));
#13420=CARTESIAN_POINT('Ctrl Pts',(29.5533069226325,177.002028447915,40.3519323616533));
#13421=CARTESIAN_POINT('Ctrl Pts',(23.1621886995185,176.502028447915,45.0327163383337));
#13422=CARTESIAN_POINT('Ctrl Pts',(15.6374322712211,176.002028447915,47.5094422967239));
#13423=CARTESIAN_POINT('Ctrl Pts',(8.11267584292359,175.502028447915,49.9861682551141));
#13424=CARTESIAN_POINT('Ctrl Pts',(0.190856796705285,175.002028447915,50.0163970020424));
#13425=CARTESIAN_POINT('Ctrl Pts',(0.000256710972400845,237.995967593475,
50.0163970020424));
#13426=CARTESIAN_POINT('Ctrl Pts',(-7.92156233524589,237.495967593475,50.0164376610661));
#13427=CARTESIAN_POINT('Ctrl Pts',(-15.4556725243922,236.995967593475,47.5684996184509));
#13428=CARTESIAN_POINT('Ctrl Pts',(-22.9897827135384,236.495967593475,45.1205615758357));
#13429=CARTESIAN_POINT('Ctrl Pts',(-29.3986928470667,235.995967593475,40.4642660629801));
#13430=CARTESIAN_POINT('Ctrl Pts',(-35.8076029805949,235.495967593475,35.8079705501245));
#13431=CARTESIAN_POINT('Ctrl Pts',(-40.4639642811328,234.995967593475,29.3991082141453));
#13432=CARTESIAN_POINT('Ctrl Pts',(-45.1203255816707,234.495967593475,22.990245878166));
#13433=CARTESIAN_POINT('Ctrl Pts',(-47.5683409623447,233.995967593475,15.4561608176784));
#13434=CARTESIAN_POINT('Ctrl Pts',(-50.0163563430187,233.495967593475,7.9220757571907));
#13435=CARTESIAN_POINT('Ctrl Pts',(-50.0163970020424,232.995967593475,0.000256710972403907));
#13436=CARTESIAN_POINT('Ctrl Pts',(-50.0164376610661,232.495967593475,-7.92156233524589));
#13437=CARTESIAN_POINT('Ctrl Pts',(-47.5684996184509,231.995967593475,-15.4556725243922));
#13438=CARTESIAN_POINT('Ctrl Pts',(-45.1205615758357,231.495967593475,-22.9897827135384));
#13439=CARTESIAN_POINT('Ctrl Pts',(-40.4642660629801,230.995967593475,-29.3986928470667));
#13440=CARTESIAN_POINT('Ctrl Pts',(-35.8079705501245,230.495967593475,-35.8076029805949));
#13441=CARTESIAN_POINT('Ctrl Pts',(-29.3991082141453,229.995967593475,-40.4639642811328));
#13442=CARTESIAN_POINT('Ctrl Pts',(-22.9902458781661,229.495967593475,-45.1203255816707));
#13443=CARTESIAN_POINT('Ctrl Pts',(-15.4561608176784,228.995967593475,-47.5683409623447));
#13444=CARTESIAN_POINT('Ctrl Pts',(-7.92207575719071,228.495967593475,-50.0163563430187));
#13445=CARTESIAN_POINT('Ctrl Pts',(-0.00025671097240697,227.995967593475,
-50.0163970020424));
#13446=CARTESIAN_POINT('Ctrl Pts',(7.92156233524589,227.495967593475,-50.0164376610661));
#13447=CARTESIAN_POINT('Ctrl Pts',(15.4556725243922,226.995967593475,-47.5684996184509));
#13448=CARTESIAN_POINT('Ctrl Pts',(22.9897827135384,226.495967593475,-45.1205615758357));
#13449=CARTESIAN_POINT('Ctrl Pts',(29.3986928470667,225.995967593475,-40.4642660629801));
#13450=CARTESIAN_POINT('Ctrl Pts',(35.8076029805949,225.495967593475,-35.8079705501245));
#13451=CARTESIAN_POINT('Ctrl Pts',(40.4639642811328,224.995967593475,-29.3991082141453));
#13452=CARTESIAN_POINT('Ctrl Pts',(45.1203255816707,224.495967593475,-22.9902458781661));
#13453=CARTESIAN_POINT('Ctrl Pts',(47.5683409623447,223.995967593475,-15.4561608176784));
#13454=CARTESIAN_POINT('Ctrl Pts',(50.0163563430187,223.495967593475,-7.92207575719071));
#13455=CARTESIAN_POINT('Ctrl Pts',(50.0163970020424,222.995967593475,-0.000256710972410033));
#13456=CARTESIAN_POINT('Ctrl Pts',(50.0164376610661,222.495967593475,7.92156233524589));
#13457=CARTESIAN_POINT('Ctrl Pts',(47.5684996184509,221.995967593475,15.4556725243922));
#13458=CARTESIAN_POINT('Ctrl Pts',(45.1205615758358,221.495967593475,22.9897827135384));
#13459=CARTESIAN_POINT('Ctrl Pts',(40.4642660629801,220.995967593475,29.3986928470667));
#13460=CARTESIAN_POINT('Ctrl Pts',(35.8079705501245,220.495967593475,35.8076029805949));
#13461=CARTESIAN_POINT('Ctrl Pts',(29.3991082141453,219.995967593475,40.4639642811328));
#13462=CARTESIAN_POINT('Ctrl Pts',(22.9902458781661,219.495967593475,45.1203255816707));
#13463=CARTESIAN_POINT('Ctrl Pts',(15.4561608176784,218.995967593475,47.5683409623447));
#13464=CARTESIAN_POINT('Ctrl Pts',(7.92207575719071,218.495967593475,50.0163563430187));
#13465=CARTESIAN_POINT('Ctrl Pts',(0.000256710972400845,217.995967593475,
50.0163970020424));
#13466=CARTESIAN_POINT('Ctrl Pts',(-7.92156233524589,217.495967593475,50.0164376610661));
#13467=CARTESIAN_POINT('Ctrl Pts',(-15.4556725243922,216.995967593475,47.5684996184509));
#13468=CARTESIAN_POINT('Ctrl Pts',(-22.9897827135384,216.495967593475,45.1205615758357));
#13469=CARTESIAN_POINT('Ctrl Pts',(-29.3986928470667,215.995967593475,40.4642660629801));
#13470=CARTESIAN_POINT('Ctrl Pts',(-35.8076029805949,215.495967593475,35.8079705501245));
#13471=CARTESIAN_POINT('Ctrl Pts',(-40.4639642811328,214.995967593475,29.3991082141453));
#13472=CARTESIAN_POINT('Ctrl Pts',(-45.1203255816707,214.495967593475,22.990245878166));
#13473=CARTESIAN_POINT('Ctrl Pts',(-47.5683409623447,213.995967593475,15.4561608176784));
#13474=CARTESIAN_POINT('Ctrl Pts',(-50.0163563430187,213.495967593475,7.9220757571907));
#13475=CARTESIAN_POINT('Ctrl Pts',(-50.0163970020424,212.995967593475,0.000256710972403907));
#13476=CARTESIAN_POINT('Ctrl Pts',(-50.0164376610661,212.495967593475,-7.92156233524589));
#13477=CARTESIAN_POINT('Ctrl Pts',(-47.5684996184509,211.995967593475,-15.4556725243922));
#13478=CARTESIAN_POINT('Ctrl Pts',(-45.1205615758357,211.495967593475,-22.9897827135384));
#13479=CARTESIAN_POINT('Ctrl Pts',(-40.4642660629801,210.995967593475,-29.3986928470667));
#13480=CARTESIAN_POINT('Ctrl Pts',(-35.8079705501245,210.495967593475,-35.8076029805949));
#13481=CARTESIAN_POINT('Ctrl Pts',(-29.3991082141453,209.995967593475,-40.4639642811328));
#13482=CARTESIAN_POINT('Ctrl Pts',(-22.9902458781661,209.495967593475,-45.1203255816707));
#13483=CARTESIAN_POINT('Ctrl Pts',(-15.4561608176784,208.995967593475,-47.5683409623447));
#13484=CARTESIAN_POINT('Ctrl Pts',(-7.92207575719071,208.495967593475,-50.0163563430187));
#13485=CARTESIAN_POINT('Ctrl Pts',(-0.00025671097240697,207.995967593475,
-50.0163970020424));
#13486=CARTESIAN_POINT('Ctrl Pts',(7.92156233524589,207.495967593475,-50.0164376610661));
#13487=CARTESIAN_POINT('Ctrl Pts',(15.4556725243922,206.995967593475,-47.5684996184509));
#13488=CARTESIAN_POINT('Ctrl Pts',(22.9897827135384,206.495967593475,-45.1205615758357));
#13489=CARTESIAN_POINT('Ctrl Pts',(29.3986928470667,205.995967593475,-40.4642660629801));
#13490=CARTESIAN_POINT('Ctrl Pts',(35.8076029805949,205.495967593475,-35.8079705501245));
#13491=CARTESIAN_POINT('Ctrl Pts',(40.4639642811328,204.995967593475,-29.3991082141453));
#13492=CARTESIAN_POINT('Ctrl Pts',(45.1203255816707,204.495967593475,-22.9902458781661));
#13493=CARTESIAN_POINT('Ctrl Pts',(47.5683409623447,203.995967593475,-15.4561608176784));
#13494=CARTESIAN_POINT('Ctrl Pts',(50.0163563430187,203.495967593475,-7.92207575719071));
#13495=CARTESIAN_POINT('Ctrl Pts',(50.0163970020424,202.995967593475,-0.000256710972410033));
#13496=CARTESIAN_POINT('Ctrl Pts',(50.0164376610661,202.495967593475,7.92156233524589));
#13497=CARTESIAN_POINT('Ctrl Pts',(47.5684996184509,201.995967593475,15.4556725243922));
#13498=CARTESIAN_POINT('Ctrl Pts',(45.1205615758358,201.495967593475,22.9897827135384));
#13499=CARTESIAN_POINT('Ctrl Pts',(40.4642660629801,200.995967593475,29.3986928470667));
#13500=CARTESIAN_POINT('Ctrl Pts',(35.8079705501245,200.495967593475,35.8076029805949));
#13501=CARTESIAN_POINT('Ctrl Pts',(29.3991082141453,199.995967593475,40.4639642811328));
#13502=CARTESIAN_POINT('Ctrl Pts',(22.9902458781661,199.495967593475,45.1203255816707));
#13503=CARTESIAN_POINT('Ctrl Pts',(15.4561608176784,198.995967593475,47.5683409623447));
#13504=CARTESIAN_POINT('Ctrl Pts',(7.92207575719071,198.495967593475,50.0163563430187));
#13505=CARTESIAN_POINT('Ctrl Pts',(0.000256710972400845,197.995967593475,
50.0163970020424));
#13506=CARTESIAN_POINT('Ctrl Pts',(-7.92156233524589,197.495967593475,50.0164376610661));
#13507=CARTESIAN_POINT('Ctrl Pts',(-15.4556725243922,196.995967593475,47.5684996184509));
#13508=CARTESIAN_POINT('Ctrl Pts',(-22.9897827135384,196.495967593475,45.1205615758357));
#13509=CARTESIAN_POINT('Ctrl Pts',(-29.3986928470667,195.995967593475,40.4642660629801));
#13510=CARTESIAN_POINT('Ctrl Pts',(-35.8076029805949,195.495967593475,35.8079705501245));
#13511=CARTESIAN_POINT('Ctrl Pts',(-40.4639642811328,194.995967593475,29.3991082141453));
#13512=CARTESIAN_POINT('Ctrl Pts',(-45.1203255816707,194.495967593475,22.990245878166));
#13513=CARTESIAN_POINT('Ctrl Pts',(-47.5683409623447,193.995967593475,15.4561608176784));
#13514=CARTESIAN_POINT('Ctrl Pts',(-50.0163563430187,193.495967593475,7.9220757571907));
#13515=CARTESIAN_POINT('Ctrl Pts',(-50.0163970020424,192.995967593475,0.000256710972403907));
#13516=CARTESIAN_POINT('Ctrl Pts',(-50.0164376610661,192.495967593475,-7.92156233524589));
#13517=CARTESIAN_POINT('Ctrl Pts',(-47.5684996184509,191.995967593475,-15.4556725243922));
#13518=CARTESIAN_POINT('Ctrl Pts',(-45.1205615758357,191.495967593475,-22.9897827135384));
#13519=CARTESIAN_POINT('Ctrl Pts',(-40.4642660629801,190.995967593475,-29.3986928470667));
#13520=CARTESIAN_POINT('Ctrl Pts',(-35.8079705501245,190.495967593475,-35.8076029805949));
#13521=CARTESIAN_POINT('Ctrl Pts',(-29.3991082141453,189.995967593475,-40.4639642811328));
#13522=CARTESIAN_POINT('Ctrl Pts',(-22.9902458781661,189.495967593475,-45.1203255816707));
#13523=CARTESIAN_POINT('Ctrl Pts',(-15.4561608176784,188.995967593475,-47.5683409623447));
#13524=CARTESIAN_POINT('Ctrl Pts',(-7.92207575719071,188.495967593475,-50.0163563430187));
#13525=CARTESIAN_POINT('Ctrl Pts',(-0.00025671097240697,187.995967593475,
-50.0163970020424));
#13526=CARTESIAN_POINT('Ctrl Pts',(7.92156233524589,187.495967593475,-50.0164376610661));
#13527=CARTESIAN_POINT('Ctrl Pts',(15.4556725243922,186.995967593475,-47.5684996184509));
#13528=CARTESIAN_POINT('Ctrl Pts',(22.9897827135384,186.495967593475,-45.1205615758357));
#13529=CARTESIAN_POINT('Ctrl Pts',(29.3986928470667,185.995967593475,-40.4642660629801));
#13530=CARTESIAN_POINT('Ctrl Pts',(35.8076029805949,185.495967593475,-35.8079705501245));
#13531=CARTESIAN_POINT('Ctrl Pts',(40.4639642811328,184.995967593475,-29.3991082141453));
#13532=CARTESIAN_POINT('Ctrl Pts',(45.1203255816707,184.495967593475,-22.9902458781661));
#13533=CARTESIAN_POINT('Ctrl Pts',(47.5683409623447,183.995967593475,-15.4561608176784));
#13534=CARTESIAN_POINT('Ctrl Pts',(50.0163563430187,183.495967593475,-7.92207575719071));
#13535=CARTESIAN_POINT('Ctrl Pts',(50.0163970020424,182.995967593475,-0.000256710972410033));
#13536=CARTESIAN_POINT('Ctrl Pts',(50.0164376610661,182.495967593475,7.92156233524589));
#13537=CARTESIAN_POINT('Ctrl Pts',(47.5684996184509,181.995967593475,15.4556725243922));
#13538=CARTESIAN_POINT('Ctrl Pts',(45.1205615758358,181.495967593475,22.9897827135384));
#13539=CARTESIAN_POINT('Ctrl Pts',(40.4642660629801,180.995967593475,29.3986928470667));
#13540=CARTESIAN_POINT('Ctrl Pts',(35.8079705501245,180.495967593475,35.8076029805949));
#13541=CARTESIAN_POINT('Ctrl Pts',(29.3991082141453,179.995967593475,40.4639642811328));
#13542=CARTESIAN_POINT('Ctrl Pts',(22.9902458781661,179.495967593475,45.1203255816707));
#13543=CARTESIAN_POINT('Ctrl Pts',(15.4561608176784,178.995967593475,47.5683409623447));
#13544=CARTESIAN_POINT('Ctrl Pts',(7.92207575719071,178.495967593475,50.0163563430187));
#13545=CARTESIAN_POINT('Ctrl Pts',(0.000256710972400845,177.995967593475,
50.0163970020424));
#13546=CARTESIAN_POINT('Origin',(0.,150.,0.));
#13547=CARTESIAN_POINT('',(-5.,100.,-24.4948974278318));
#13548=CARTESIAN_POINT('',(5.,100.,-24.4948974278318));
#13549=CARTESIAN_POINT('Origin',(0.,100.,0.));
#13550=CARTESIAN_POINT('',(5.,150.,-24.4948974278318));
#13551=CARTESIAN_POINT('',(5.,150.,-24.4948974278318));
#13552=CARTESIAN_POINT('',(-5.,150.,-24.4948974278318));
#13553=CARTESIAN_POINT('Origin',(0.,150.,0.));
#13554=CARTESIAN_POINT('',(-5.,150.,-24.4948974278318));
#13555=CARTESIAN_POINT('Origin',(5.,150.,-33.));
#13556=CARTESIAN_POINT('',(5.,100.,-33.));
#13557=CARTESIAN_POINT('',(5.,100.,-24.4948974278318));
#13558=CARTESIAN_POINT('',(5.,150.,-33.));
#13559=CARTESIAN_POINT('',(5.,150.,-33.));
#13560=CARTESIAN_POINT('',(5.,150.,-24.4948974278318));
#13561=CARTESIAN_POINT('Origin',(-5.,150.,-33.));
#13562=CARTESIAN_POINT('',(-5.,100.,-33.));
#13563=CARTESIAN_POINT('',(5.,100.,-33.));
#13564=CARTESIAN_POINT('',(-5.,150.,-33.));
#13565=CARTESIAN_POINT('',(-5.,150.,-33.));
#13566=CARTESIAN_POINT('',(5.,150.,-33.));
#13567=CARTESIAN_POINT('Origin',(-5.,150.,-33.));
#13568=CARTESIAN_POINT('',(-5.,100.,-33.));
#13569=CARTESIAN_POINT('',(-5.,150.,-33.));
#13570=CARTESIAN_POINT('Origin',(0.,150.,0.));
#13571=CARTESIAN_POINT('Origin',(0.,100.,0.));
#13584=UNCERTAINTY_MEASURE_WITH_UNIT(LENGTH_MEASURE(0.01),#13595,
'DISTANCE_ACCURACY_VALUE',
'Maximum model space distance between geometric entities at asserted c
onnectivities');
#13585=UNCERTAINTY_MEASURE_WITH_UNIT(LENGTH_MEASURE(0.01),#13595,
'DISTANCE_ACCURACY_VALUE',
'Maximum model space distance between geometric entities at asserted c
onnectivities');
#13593=(
GEOMETRIC_REPRESENTATION_CONTEXT(3)
GLOBAL_UNCERTAINTY_ASSIGNED_CONTEXT((#13584))
GLOBAL_UNIT_ASSIGNED_CONTEXT((#13595,#13597,#13598))
REPRESENTATION_CONTEXT('','3D')
);
#13594=(
GEOMETRIC_REPRESENTATION_CONTEXT(3)
GLOBAL_UNCERTAINTY_ASSIGNED_CONTEXT((#13585))
GLOBAL_UNIT_ASSIGNED_CONTEXT((#13595,#13597,#13598))
REPRESENTATION_CONTEXT('','3D')
);
#13595=(
LENGTH_UNIT()
NAMED_UNIT(*)
SI_UNIT(.MILLI.,.METRE.)
);
#13597=(
NAMED_UNIT(*)
PLANE_ANGLE_UNIT()
SI_UNIT($,.RADIAN.)
);
#13598=(
NAMED_UNIT(*)
SI_UNIT($,.STERADIAN.)
SOLID_ANGLE_UNIT()
);
#13606=SHAPE_DEFINITION_REPRESENTATION(#13617,#13630);
#13617=PRODUCT_DEFINITION_SHAPE('',$,#13639);
#13630=SHAPE_REPRESENTATION('',(#3252),#13593);
#13631=PRODUCT_DEFINITION_CONTEXT('part definition',#13657,'design');
#13639=PRODUCT_DEFINITION('Screw Feeder','Screw Feeder',#13647,#13631);
#13647=PRODUCT_DEFINITION_FORMATION('',$,#13666);
#13657=APPLICATION_CONTEXT(
'Core Data for Automotive Mechanical Design Process');
#13658=PRODUCT_CONTEXT('part definition',#13657,'mechanical');
#13666=PRODUCT('Screw Feeder','Screw Feeder',$,(#13658));
#13667=PRESENTATION_STYLE_ASSIGNMENT((#13668));
#13668=SURFACE_STYLE_USAGE(.BOTH.,#13669);
#13669=SURFACE_SIDE_STYLE('',(#13670));
#13670=SURFACE_STYLE_FILL_AREA(#13671);
#13671=FILL_AREA_STYLE('Steel - Satin',(#13672));
#13672=FILL_AREA_STYLE_COLOUR('Steel - Satin',#13673);
#13673=COLOUR_RGB('Steel - Satin',0.627450980392157,0.627450980392157,0.627450980392157);
ENDSEC;
END-ISO-10303-21;
